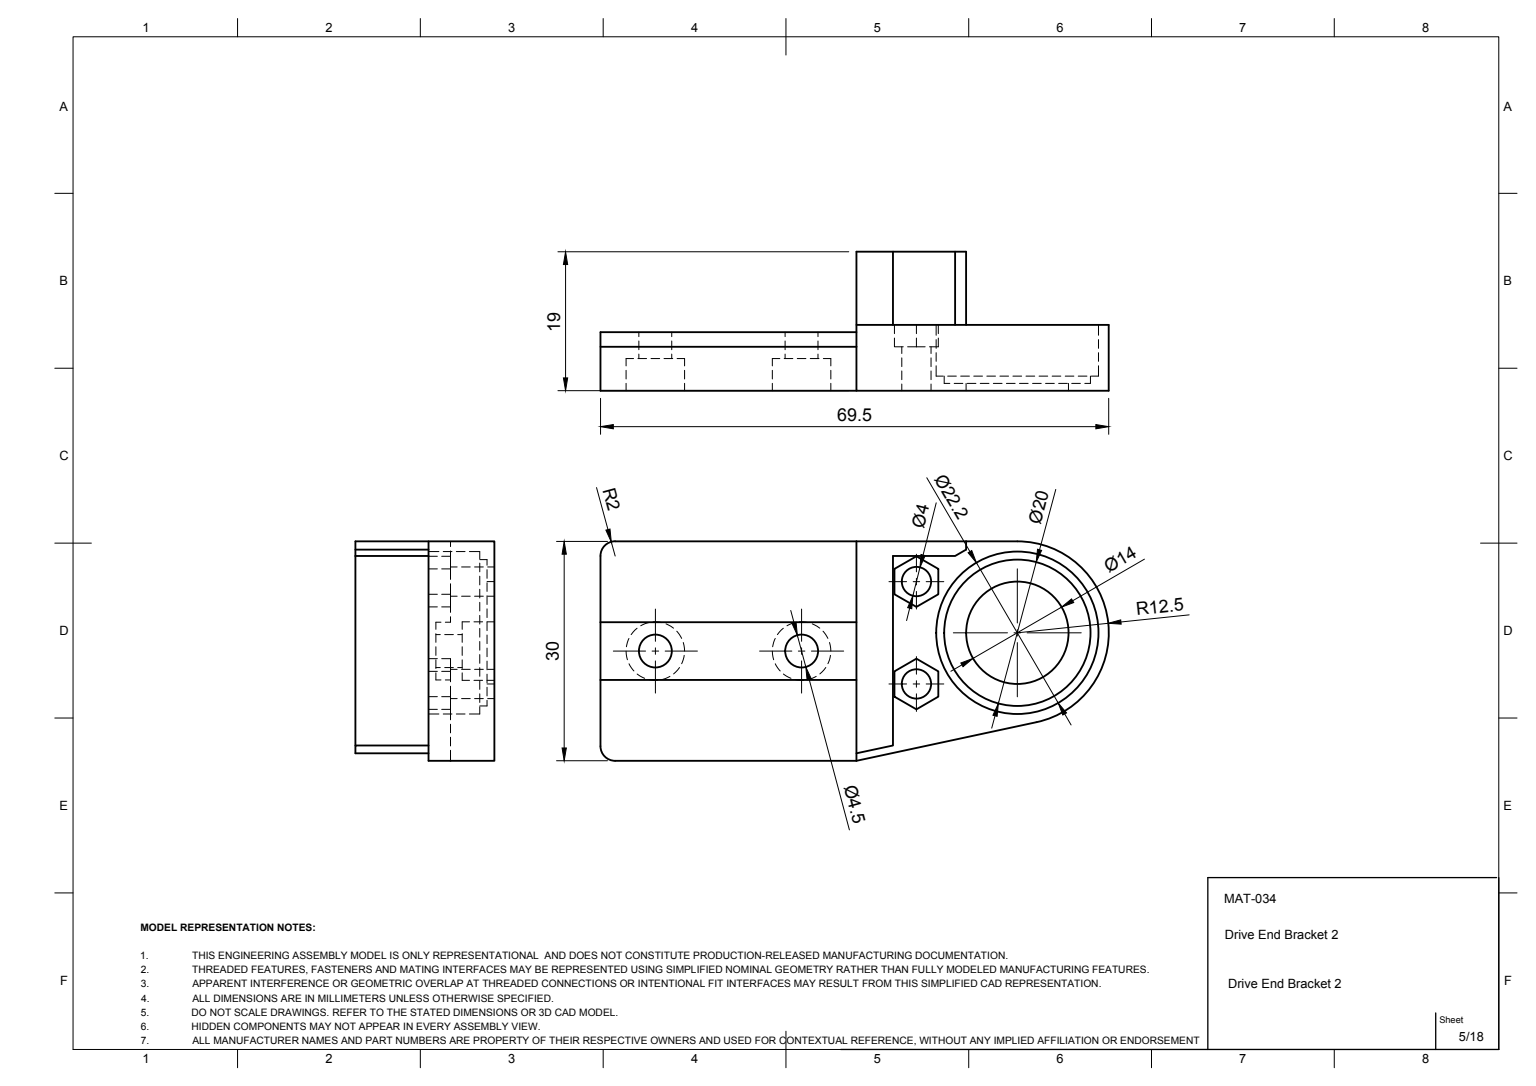
ISO-10303-21;
HEADER;
/* Generated by software containing ST-Developer
 * from STEP Tools, Inc. (www.steptools.com) 
 */

FILE_DESCRIPTION(
/* description */ ('STEP AP214'),
/* implementation_level */ '2;1');

FILE_NAME(
/* name */ 'Drive End Bracket 2.step',
/* time_stamp */ '2026-11-14T09:24:36-08:00',
/* author */ (''),
/* organization */ (''),
/* preprocessor_version */ 'ST-DEVELOPER v20.2',
/* originating_system */ 'Autodesk Translation Framework v15.17.0.0',
/* authorisation */ '');

FILE_SCHEMA (('AUTOMOTIVE_DESIGN { 1 0 10303 214 3 1 1 }'));
ENDSEC;

DATA;
#10=MECHANICAL_DESIGN_GEOMETRIC_PRESENTATION_REPRESENTATION('',(#204),#18867);
#172=SHAPE_REPRESENTATION_RELATIONSHIP('SRR','None',#18936,#188);
#188=ADVANCED_BREP_SHAPE_REPRESENTATION('',(#228),#18852);
#204=STYLED_ITEM('',(#19024),#228);
#228=MANIFOLD_SOLID_BREP('Body1',#10959);
#267=FACE_BOUND('',#1398,.T.);
#268=FACE_BOUND('',#1399,.T.);
#269=FACE_BOUND('',#1400,.T.);
#270=FACE_BOUND('',#1407,.T.);
#271=FACE_BOUND('',#1408,.T.);
#272=FACE_BOUND('',#1409,.T.);
#273=FACE_BOUND('',#1410,.T.);
#274=FACE_BOUND('',#1411,.T.);
#275=FACE_BOUND('',#1413,.T.);
#276=FACE_BOUND('',#1415,.T.);
#277=FACE_BOUND('',#1422,.T.);
#278=FACE_BOUND('',#1424,.T.);
#279=FACE_BOUND('',#1432,.T.);
#280=FACE_BOUND('',#1440,.T.);
#281=FACE_BOUND('',#1445,.T.);
#282=FACE_BOUND('',#1446,.T.);
#417=PLANE('',#11261);
#418=PLANE('',#11262);
#419=PLANE('',#11264);
#420=PLANE('',#11266);
#421=PLANE('',#11268);
#422=PLANE('',#11271);
#423=PLANE('',#11272);
#424=PLANE('',#11273);
#425=PLANE('',#11274);
#426=PLANE('',#11277);
#427=PLANE('',#11278);
#428=PLANE('',#11279);
#429=PLANE('',#11280);
#430=PLANE('',#11281);
#431=PLANE('',#11284);
#432=PLANE('',#11285);
#433=PLANE('',#11286);
#434=PLANE('',#11287);
#435=PLANE('',#11288);
#436=PLANE('',#11289);
#437=PLANE('',#11290);
#438=PLANE('',#11291);
#439=PLANE('',#11292);
#440=PLANE('',#11293);
#441=PLANE('',#11294);
#442=PLANE('',#11295);
#443=PLANE('',#11296);
#444=PLANE('',#11297);
#445=PLANE('',#11298);
#446=PLANE('',#11299);
#447=PLANE('',#11300);
#448=PLANE('',#11301);
#449=PLANE('',#11302);
#450=PLANE('',#11303);
#451=PLANE('',#11304);
#452=PLANE('',#11305);
#773=FACE_OUTER_BOUND('',#1385,.T.);
#774=FACE_OUTER_BOUND('',#1386,.T.);
#775=FACE_OUTER_BOUND('',#1387,.T.);
#776=FACE_OUTER_BOUND('',#1388,.T.);
#777=FACE_OUTER_BOUND('',#1389,.T.);
#778=FACE_OUTER_BOUND('',#1390,.T.);
#779=FACE_OUTER_BOUND('',#1391,.T.);
#780=FACE_OUTER_BOUND('',#1392,.T.);
#781=FACE_OUTER_BOUND('',#1393,.T.);
#782=FACE_OUTER_BOUND('',#1394,.T.);
#783=FACE_OUTER_BOUND('',#1395,.T.);
#784=FACE_OUTER_BOUND('',#1396,.T.);
#785=FACE_OUTER_BOUND('',#1397,.T.);
#786=FACE_OUTER_BOUND('',#1401,.T.);
#787=FACE_OUTER_BOUND('',#1402,.T.);
#788=FACE_OUTER_BOUND('',#1403,.T.);
#789=FACE_OUTER_BOUND('',#1404,.T.);
#790=FACE_OUTER_BOUND('',#1405,.T.);
#791=FACE_OUTER_BOUND('',#1406,.T.);
#792=FACE_OUTER_BOUND('',#1412,.T.);
#793=FACE_OUTER_BOUND('',#1414,.T.);
#794=FACE_OUTER_BOUND('',#1416,.T.);
#795=FACE_OUTER_BOUND('',#1417,.T.);
#796=FACE_OUTER_BOUND('',#1418,.T.);
#797=FACE_OUTER_BOUND('',#1419,.T.);
#798=FACE_OUTER_BOUND('',#1420,.T.);
#799=FACE_OUTER_BOUND('',#1421,.T.);
#800=FACE_OUTER_BOUND('',#1423,.T.);
#801=FACE_OUTER_BOUND('',#1425,.T.);
#802=FACE_OUTER_BOUND('',#1426,.T.);
#803=FACE_OUTER_BOUND('',#1427,.T.);
#804=FACE_OUTER_BOUND('',#1428,.T.);
#805=FACE_OUTER_BOUND('',#1429,.T.);
#806=FACE_OUTER_BOUND('',#1430,.T.);
#807=FACE_OUTER_BOUND('',#1431,.T.);
#808=FACE_OUTER_BOUND('',#1433,.T.);
#809=FACE_OUTER_BOUND('',#1434,.T.);
#810=FACE_OUTER_BOUND('',#1435,.T.);
#811=FACE_OUTER_BOUND('',#1436,.T.);
#812=FACE_OUTER_BOUND('',#1437,.T.);
#813=FACE_OUTER_BOUND('',#1438,.T.);
#814=FACE_OUTER_BOUND('',#1439,.T.);
#815=FACE_OUTER_BOUND('',#1441,.T.);
#816=FACE_OUTER_BOUND('',#1442,.T.);
#817=FACE_OUTER_BOUND('',#1443,.T.);
#818=FACE_OUTER_BOUND('',#1444,.T.);
#819=FACE_OUTER_BOUND('',#1447,.T.);
#820=FACE_OUTER_BOUND('',#1448,.T.);
#1385=EDGE_LOOP('',(#7346,#7347,#7348,#7349));
#1386=EDGE_LOOP('',(#7350,#7351,#7352,#7353));
#1387=EDGE_LOOP('',(#7354,#7355,#7356,#7357));
#1388=EDGE_LOOP('',(#7358,#7359,#7360,#7361));
#1389=EDGE_LOOP('',(#7362,#7363,#7364,#7365));
#1390=EDGE_LOOP('',(#7366,#7367,#7368,#7369));
#1391=EDGE_LOOP('',(#7370,#7371,#7372,#7373));
#1392=EDGE_LOOP('',(#7374,#7375,#7376,#7377));
#1393=EDGE_LOOP('',(#7378,#7379,#7380,#7381));
#1394=EDGE_LOOP('',(#7382,#7383,#7384,#7385,#7386,#7387,#7388,#7389,#7390,
#7391));
#1395=EDGE_LOOP('',(#7392,#7393,#7394,#7395,#7396));
#1396=EDGE_LOOP('',(#7397,#7398,#7399,#7400,#7401));
#1397=EDGE_LOOP('',(#7402,#7403,#7404,#7405,#7406,#7407,#7408,#7409,#7410));
#1398=EDGE_LOOP('',(#7411,#7412,#7413,#7414,#7415,#7416));
#1399=EDGE_LOOP('',(#7417,#7418,#7419,#7420,#7421,#7422));
#1400=EDGE_LOOP('',(#7423));
#1401=EDGE_LOOP('',(#7424,#7425,#7426,#7427,#7428));
#1402=EDGE_LOOP('',(#7429,#7430,#7431,#7432));
#1403=EDGE_LOOP('',(#7433,#7434,#7435,#7436,#7437,#7438,#7439,#7440));
#1404=EDGE_LOOP('',(#7441,#7442,#7443,#7444,#7445,#7446,#7447,#7448));
#1405=EDGE_LOOP('',(#7449,#7450,#7451,#7452));
#1406=EDGE_LOOP('',(#7453,#7454,#7455,#7456,#7457,#7458,#7459));
#1407=EDGE_LOOP('',(#7460));
#1408=EDGE_LOOP('',(#7461));
#1409=EDGE_LOOP('',(#7462));
#1410=EDGE_LOOP('',(#7463));
#1411=EDGE_LOOP('',(#7464));
#1412=EDGE_LOOP('',(#7465));
#1413=EDGE_LOOP('',(#7466));
#1414=EDGE_LOOP('',(#7467));
#1415=EDGE_LOOP('',(#7468));
#1416=EDGE_LOOP('',(#7469,#7470,#7471,#7472));
#1417=EDGE_LOOP('',(#7473,#7474,#7475,#7476));
#1418=EDGE_LOOP('',(#7477,#7478,#7479,#7480,#7481,#7482,#7483));
#1419=EDGE_LOOP('',(#7484,#7485,#7486,#7487));
#1420=EDGE_LOOP('',(#7488,#7489,#7490,#7491));
#1421=EDGE_LOOP('',(#7492));
#1422=EDGE_LOOP('',(#7493));
#1423=EDGE_LOOP('',(#7494));
#1424=EDGE_LOOP('',(#7495));
#1425=EDGE_LOOP('',(#7496,#7497,#7498,#7499));
#1426=EDGE_LOOP('',(#7500,#7501,#7502,#7503));
#1427=EDGE_LOOP('',(#7504,#7505,#7506,#7507));
#1428=EDGE_LOOP('',(#7508,#7509,#7510,#7511));
#1429=EDGE_LOOP('',(#7512,#7513,#7514,#7515));
#1430=EDGE_LOOP('',(#7516,#7517,#7518,#7519));
#1431=EDGE_LOOP('',(#7520,#7521,#7522,#7523,#7524,#7525));
#1432=EDGE_LOOP('',(#7526));
#1433=EDGE_LOOP('',(#7527,#7528,#7529,#7530));
#1434=EDGE_LOOP('',(#7531,#7532,#7533,#7534));
#1435=EDGE_LOOP('',(#7535,#7536,#7537,#7538));
#1436=EDGE_LOOP('',(#7539,#7540,#7541,#7542));
#1437=EDGE_LOOP('',(#7543,#7544,#7545,#7546));
#1438=EDGE_LOOP('',(#7547,#7548,#7549,#7550));
#1439=EDGE_LOOP('',(#7551,#7552,#7553,#7554,#7555,#7556));
#1440=EDGE_LOOP('',(#7557));
#1441=EDGE_LOOP('',(#7558,#7559,#7560,#7561));
#1442=EDGE_LOOP('',(#7562,#7563,#7564,#7565));
#1443=EDGE_LOOP('',(#7566,#7567,#7568,#7569));
#1444=EDGE_LOOP('',(#7570,#7571,#7572,#7573));
#1445=EDGE_LOOP('',(#7574));
#1446=EDGE_LOOP('',(#7575));
#1447=EDGE_LOOP('',(#7576,#7577,#7578,#7579));
#1448=EDGE_LOOP('',(#7580,#7581,#7582,#7583));
#2142=LINE('',#15858,#3156);
#2143=LINE('',#15864,#3157);
#2144=LINE('',#15870,#3158);
#2145=LINE('',#15876,#3159);
#2146=LINE('',#15882,#3160);
#2147=LINE('',#15888,#3161);
#2148=LINE('',#15894,#3162);
#2149=LINE('',#15900,#3163);
#2150=LINE('',#15906,#3164);
#2151=LINE('',#15911,#3165);
#2152=LINE('',#15913,#3166);
#2153=LINE('',#15915,#3167);
#2154=LINE('',#15917,#3168);
#2155=LINE('',#15919,#3169);
#2156=LINE('',#15921,#3170);
#2157=LINE('',#15923,#3171);
#2158=LINE('',#15925,#3172);
#2159=LINE('',#15927,#3173);
#2160=LINE('',#15928,#3174);
#2161=LINE('',#15931,#3175);
#2162=LINE('',#15933,#3176);
#2163=LINE('',#15936,#3177);
#2164=LINE('',#15939,#3178);
#2165=LINE('',#15941,#3179);
#2166=LINE('',#15944,#3180);
#2167=LINE('',#15948,#3181);
#2168=LINE('',#15950,#3182);
#2169=LINE('',#15951,#3183);
#2170=LINE('',#15953,#3184);
#2171=LINE('',#15957,#3185);
#2172=LINE('',#15959,#3186);
#2173=LINE('',#15960,#3187);
#2174=LINE('',#15963,#3188);
#2175=LINE('',#15965,#3189);
#2176=LINE('',#15967,#3190);
#2177=LINE('',#15969,#3191);
#2178=LINE('',#15971,#3192);
#2179=LINE('',#15972,#3193);
#2180=LINE('',#15975,#3194);
#2181=LINE('',#15977,#3195);
#2182=LINE('',#15979,#3196);
#2183=LINE('',#15981,#3197);
#2184=LINE('',#15983,#3198);
#2185=LINE('',#15984,#3199);
#2186=LINE('',#15987,#3200);
#2187=LINE('',#15989,#3201);
#2188=LINE('',#15990,#3202);
#2189=LINE('',#15994,#3203);
#2190=LINE('',#15997,#3204);
#2191=LINE('',#15998,#3205);
#2192=LINE('',#16000,#3206);
#2193=LINE('',#16001,#3207);
#2194=LINE('',#16004,#3208);
#2195=LINE('',#16006,#3209);
#2196=LINE('',#16007,#3210);
#2197=LINE('',#16009,#3211);
#2198=LINE('',#16011,#3212);
#2199=LINE('',#16012,#3213);
#2200=LINE('',#16015,#3214);
#2201=LINE('',#16016,#3215);
#2202=LINE('',#16024,#3216);
#2203=LINE('',#16025,#3217);
#2204=LINE('',#16028,#3218);
#2205=LINE('',#16029,#3219);
#2206=LINE('',#16032,#3220);
#2207=LINE('',#16034,#3221);
#2208=LINE('',#16035,#3222);
#2209=LINE('',#16042,#3223);
#2210=LINE('',#16044,#3224);
#2211=LINE('',#16045,#3225);
#2212=LINE('',#16048,#3226);
#2213=LINE('',#16049,#3227);
#2214=LINE('',#16052,#3228);
#2215=LINE('',#16053,#3229);
#2216=LINE('',#16056,#3230);
#2217=LINE('',#16057,#3231);
#2218=LINE('',#16060,#3232);
#2219=LINE('',#16061,#3233);
#2220=LINE('',#16063,#3234);
#2221=LINE('',#16067,#3235);
#2222=LINE('',#16069,#3236);
#2223=LINE('',#16070,#3237);
#2224=LINE('',#16073,#3238);
#2225=LINE('',#16074,#3239);
#2226=LINE('',#16077,#3240);
#2227=LINE('',#16078,#3241);
#2228=LINE('',#16081,#3242);
#2229=LINE('',#16082,#3243);
#2230=LINE('',#16085,#3244);
#2231=LINE('',#16086,#3245);
#2232=LINE('',#16088,#3246);
#2233=LINE('',#16091,#3247);
#2234=LINE('',#16093,#3248);
#2235=LINE('',#16096,#3249);
#2236=LINE('',#16097,#3250);
#3156=VECTOR('',#12552,2.);
#3157=VECTOR('',#12559,2.);
#3158=VECTOR('',#12566,4.);
#3159=VECTOR('',#12573,2.25);
#3160=VECTOR('',#12580,4.);
#3161=VECTOR('',#12587,2.25);
#3162=VECTOR('',#12594,7.00000000000001);
#3163=VECTOR('',#12601,10.);
#3164=VECTOR('',#12608,11.1);
#3165=VECTOR('',#12613,1000.);
#3166=VECTOR('',#12614,1000.);
#3167=VECTOR('',#12615,1000.);
#3168=VECTOR('',#12616,1000.);
#3169=VECTOR('',#12617,1000.);
#3170=VECTOR('',#12618,1000.);
#3171=VECTOR('',#12619,1000.);
#3172=VECTOR('',#12620,1000.);
#3173=VECTOR('',#12621,1000.);
#3174=VECTOR('',#12622,1000.);
#3175=VECTOR('',#12625,1000.);
#3176=VECTOR('',#12626,1000.);
#3177=VECTOR('',#12629,1000.);
#3178=VECTOR('',#12632,1000.);
#3179=VECTOR('',#12633,1000.);
#3180=VECTOR('',#12636,1000.);
#3181=VECTOR('',#12639,1000.);
#3182=VECTOR('',#12640,1000.);
#3183=VECTOR('',#12641,1000.);
#3184=VECTOR('',#12642,1000.);
#3185=VECTOR('',#12645,1000.);
#3186=VECTOR('',#12646,1000.);
#3187=VECTOR('',#12647,1000.);
#3188=VECTOR('',#12648,1000.);
#3189=VECTOR('',#12649,1000.);
#3190=VECTOR('',#12650,1000.);
#3191=VECTOR('',#12651,1000.);
#3192=VECTOR('',#12652,1000.);
#3193=VECTOR('',#12653,1000.);
#3194=VECTOR('',#12654,1000.);
#3195=VECTOR('',#12655,1000.);
#3196=VECTOR('',#12656,1000.);
#3197=VECTOR('',#12657,1000.);
#3198=VECTOR('',#12658,1000.);
#3199=VECTOR('',#12659,1000.);
#3200=VECTOR('',#12662,1000.);
#3201=VECTOR('',#12663,1000.);
#3202=VECTOR('',#12664,1000.);
#3203=VECTOR('',#12669,1000.);
#3204=VECTOR('',#12672,1000.);
#3205=VECTOR('',#12673,1000.);
#3206=VECTOR('',#12674,1000.);
#3207=VECTOR('',#12675,1000.);
#3208=VECTOR('',#12678,1000.);
#3209=VECTOR('',#12679,1000.);
#3210=VECTOR('',#12680,1000.);
#3211=VECTOR('',#12681,1000.);
#3212=VECTOR('',#12682,1000.);
#3213=VECTOR('',#12683,1000.);
#3214=VECTOR('',#12686,1000.);
#3215=VECTOR('',#12687,1000.);
#3216=VECTOR('',#12700,1000.);
#3217=VECTOR('',#12701,1000.);
#3218=VECTOR('',#12704,1000.);
#3219=VECTOR('',#12705,1000.);
#3220=VECTOR('',#12708,1000.);
#3221=VECTOR('',#12709,1000.);
#3222=VECTOR('',#12710,1000.);
#3223=VECTOR('',#12721,1000.);
#3224=VECTOR('',#12722,1000.);
#3225=VECTOR('',#12723,1000.);
#3226=VECTOR('',#12726,1000.);
#3227=VECTOR('',#12727,1000.);
#3228=VECTOR('',#12730,1000.);
#3229=VECTOR('',#12731,1000.);
#3230=VECTOR('',#12734,1000.);
#3231=VECTOR('',#12735,1000.);
#3232=VECTOR('',#12738,1000.);
#3233=VECTOR('',#12739,1000.);
#3234=VECTOR('',#12742,1000.);
#3235=VECTOR('',#12747,1000.);
#3236=VECTOR('',#12748,1000.);
#3237=VECTOR('',#12749,1000.);
#3238=VECTOR('',#12752,1000.);
#3239=VECTOR('',#12753,1000.);
#3240=VECTOR('',#12756,1000.);
#3241=VECTOR('',#12757,1000.);
#3242=VECTOR('',#12760,1000.);
#3243=VECTOR('',#12761,1000.);
#3244=VECTOR('',#12764,1000.);
#3245=VECTOR('',#12765,1000.);
#3246=VECTOR('',#12768,1000.);
#3247=VECTOR('',#12773,1000.);
#3248=VECTOR('',#12776,1000.);
#3249=VECTOR('',#12781,1000.);
#3250=VECTOR('',#12782,1000.);
#4099=CIRCLE('',#11235,2.);
#4100=CIRCLE('',#11236,2.);
#4101=CIRCLE('',#11238,2.);
#4102=CIRCLE('',#11239,2.);
#4103=CIRCLE('',#11241,4.);
#4104=CIRCLE('',#11242,4.);
#4105=CIRCLE('',#11244,2.25000000000001);
#4106=CIRCLE('',#11245,2.25);
#4107=CIRCLE('',#11247,4.);
#4108=CIRCLE('',#11248,4.);
#4109=CIRCLE('',#11250,2.25000000000001);
#4110=CIRCLE('',#11251,2.25);
#4111=CIRCLE('',#11253,7.00000000000001);
#4112=CIRCLE('',#11254,7.00000000000001);
#4113=CIRCLE('',#11256,10.);
#4114=CIRCLE('',#11257,10.);
#4115=CIRCLE('',#11259,11.1);
#4116=CIRCLE('',#11260,11.1);
#4117=CIRCLE('',#11263,2.);
#4118=CIRCLE('',#11265,2.);
#4119=CIRCLE('',#11267,12.5);
#4120=CIRCLE('',#11270,12.5);
#4121=CIRCLE('',#11275,2.);
#4122=CIRCLE('',#11276,2.);
#4653=VERTEX_POINT('',#15855);
#4654=VERTEX_POINT('',#15857);
#4655=VERTEX_POINT('',#15861);
#4656=VERTEX_POINT('',#15863);
#4657=VERTEX_POINT('',#15867);
#4658=VERTEX_POINT('',#15869);
#4659=VERTEX_POINT('',#15873);
#4660=VERTEX_POINT('',#15875);
#4661=VERTEX_POINT('',#15879);
#4662=VERTEX_POINT('',#15881);
#4663=VERTEX_POINT('',#15885);
#4664=VERTEX_POINT('',#15887);
#4665=VERTEX_POINT('',#15891);
#4666=VERTEX_POINT('',#15893);
#4667=VERTEX_POINT('',#15897);
#4668=VERTEX_POINT('',#15899);
#4669=VERTEX_POINT('',#15903);
#4670=VERTEX_POINT('',#15905);
#4671=VERTEX_POINT('',#15909);
#4672=VERTEX_POINT('',#15910);
#4673=VERTEX_POINT('',#15912);
#4674=VERTEX_POINT('',#15914);
#4675=VERTEX_POINT('',#15916);
#4676=VERTEX_POINT('',#15918);
#4677=VERTEX_POINT('',#15920);
#4678=VERTEX_POINT('',#15922);
#4679=VERTEX_POINT('',#15924);
#4680=VERTEX_POINT('',#15926);
#4681=VERTEX_POINT('',#15930);
#4682=VERTEX_POINT('',#15932);
#4683=VERTEX_POINT('',#15934);
#4684=VERTEX_POINT('',#15938);
#4685=VERTEX_POINT('',#15940);
#4686=VERTEX_POINT('',#15942);
#4687=VERTEX_POINT('',#15946);
#4688=VERTEX_POINT('',#15947);
#4689=VERTEX_POINT('',#15949);
#4690=VERTEX_POINT('',#15952);
#4691=VERTEX_POINT('',#15954);
#4692=VERTEX_POINT('',#15956);
#4693=VERTEX_POINT('',#15958);
#4694=VERTEX_POINT('',#15961);
#4695=VERTEX_POINT('',#15962);
#4696=VERTEX_POINT('',#15964);
#4697=VERTEX_POINT('',#15966);
#4698=VERTEX_POINT('',#15968);
#4699=VERTEX_POINT('',#15970);
#4700=VERTEX_POINT('',#15973);
#4701=VERTEX_POINT('',#15974);
#4702=VERTEX_POINT('',#15976);
#4703=VERTEX_POINT('',#15978);
#4704=VERTEX_POINT('',#15980);
#4705=VERTEX_POINT('',#15982);
#4706=VERTEX_POINT('',#15986);
#4707=VERTEX_POINT('',#15988);
#4708=VERTEX_POINT('',#15992);
#4709=VERTEX_POINT('',#15996);
#4710=VERTEX_POINT('',#15999);
#4711=VERTEX_POINT('',#16003);
#4712=VERTEX_POINT('',#16005);
#4713=VERTEX_POINT('',#16008);
#4714=VERTEX_POINT('',#16010);
#4715=VERTEX_POINT('',#16014);
#4716=VERTEX_POINT('',#16023);
#4717=VERTEX_POINT('',#16027);
#4718=VERTEX_POINT('',#16031);
#4719=VERTEX_POINT('',#16033);
#4720=VERTEX_POINT('',#16041);
#4721=VERTEX_POINT('',#16043);
#4722=VERTEX_POINT('',#16047);
#4723=VERTEX_POINT('',#16051);
#4724=VERTEX_POINT('',#16055);
#4725=VERTEX_POINT('',#16059);
#4726=VERTEX_POINT('',#16066);
#4727=VERTEX_POINT('',#16068);
#4728=VERTEX_POINT('',#16072);
#4729=VERTEX_POINT('',#16076);
#4730=VERTEX_POINT('',#16080);
#4731=VERTEX_POINT('',#16084);
#5706=EDGE_CURVE('',#4653,#4653,#4099,.T.);
#5707=EDGE_CURVE('',#4653,#4654,#2142,.T.);
#5708=EDGE_CURVE('',#4654,#4654,#4100,.T.);
#5709=EDGE_CURVE('',#4655,#4655,#4101,.T.);
#5710=EDGE_CURVE('',#4655,#4656,#2143,.T.);
#5711=EDGE_CURVE('',#4656,#4656,#4102,.T.);
#5712=EDGE_CURVE('',#4657,#4657,#4103,.T.);
#5713=EDGE_CURVE('',#4657,#4658,#2144,.T.);
#5714=EDGE_CURVE('',#4658,#4658,#4104,.T.);
#5715=EDGE_CURVE('',#4659,#4659,#4105,.T.);
#5716=EDGE_CURVE('',#4659,#4660,#2145,.T.);
#5717=EDGE_CURVE('',#4660,#4660,#4106,.T.);
#5718=EDGE_CURVE('',#4661,#4661,#4107,.T.);
#5719=EDGE_CURVE('',#4661,#4662,#2146,.T.);
#5720=EDGE_CURVE('',#4662,#4662,#4108,.T.);
#5721=EDGE_CURVE('',#4663,#4663,#4109,.T.);
#5722=EDGE_CURVE('',#4663,#4664,#2147,.T.);
#5723=EDGE_CURVE('',#4664,#4664,#4110,.T.);
#5724=EDGE_CURVE('',#4665,#4665,#4111,.T.);
#5725=EDGE_CURVE('',#4665,#4666,#2148,.T.);
#5726=EDGE_CURVE('',#4666,#4666,#4112,.T.);
#5727=EDGE_CURVE('',#4667,#4667,#4113,.T.);
#5728=EDGE_CURVE('',#4667,#4668,#2149,.T.);
#5729=EDGE_CURVE('',#4668,#4668,#4114,.T.);
#5730=EDGE_CURVE('',#4669,#4669,#4115,.T.);
#5731=EDGE_CURVE('',#4669,#4670,#2150,.T.);
#5732=EDGE_CURVE('',#4670,#4670,#4116,.T.);
#5733=EDGE_CURVE('',#4671,#4672,#2151,.T.);
#5734=EDGE_CURVE('',#4673,#4672,#2152,.T.);
#5735=EDGE_CURVE('',#4674,#4673,#2153,.T.);
#5736=EDGE_CURVE('',#4674,#4675,#2154,.T.);
#5737=EDGE_CURVE('',#4676,#4675,#2155,.T.);
#5738=EDGE_CURVE('',#4676,#4677,#2156,.T.);
#5739=EDGE_CURVE('',#4678,#4677,#2157,.T.);
#5740=EDGE_CURVE('',#4679,#4678,#2158,.T.);
#5741=EDGE_CURVE('',#4680,#4679,#2159,.T.);
#5742=EDGE_CURVE('',#4680,#4671,#2160,.T.);
#5743=EDGE_CURVE('',#4672,#4681,#2161,.T.);
#5744=EDGE_CURVE('',#4682,#4681,#2162,.T.);
#5745=EDGE_CURVE('',#4683,#4682,#4117,.T.);
#5746=EDGE_CURVE('',#4673,#4683,#2163,.T.);
#5747=EDGE_CURVE('',#4684,#4679,#2164,.T.);
#5748=EDGE_CURVE('',#4678,#4685,#2165,.T.);
#5749=EDGE_CURVE('',#4686,#4685,#4118,.T.);
#5750=EDGE_CURVE('',#4684,#4686,#2166,.T.);
#5751=EDGE_CURVE('',#4687,#4688,#2167,.T.);
#5752=EDGE_CURVE('',#4687,#4689,#2168,.T.);
#5753=EDGE_CURVE('',#4689,#4675,#2169,.T.);
#5754=EDGE_CURVE('',#4690,#4674,#2170,.T.);
#5755=EDGE_CURVE('',#4690,#4691,#4119,.T.);
#5756=EDGE_CURVE('',#4692,#4691,#2171,.T.);
#5757=EDGE_CURVE('',#4693,#4692,#2172,.T.);
#5758=EDGE_CURVE('',#4688,#4693,#2173,.T.);
#5759=EDGE_CURVE('',#4694,#4695,#2174,.T.);
#5760=EDGE_CURVE('',#4695,#4696,#2175,.T.);
#5761=EDGE_CURVE('',#4696,#4697,#2176,.T.);
#5762=EDGE_CURVE('',#4697,#4698,#2177,.T.);
#5763=EDGE_CURVE('',#4698,#4699,#2178,.T.);
#5764=EDGE_CURVE('',#4699,#4694,#2179,.T.);
#5765=EDGE_CURVE('',#4700,#4701,#2180,.T.);
#5766=EDGE_CURVE('',#4701,#4702,#2181,.T.);
#5767=EDGE_CURVE('',#4702,#4703,#2182,.T.);
#5768=EDGE_CURVE('',#4703,#4704,#2183,.T.);
#5769=EDGE_CURVE('',#4704,#4705,#2184,.T.);
#5770=EDGE_CURVE('',#4705,#4700,#2185,.T.);
#5771=EDGE_CURVE('',#4706,#4673,#2186,.T.);
#5772=EDGE_CURVE('',#4707,#4706,#2187,.T.);
#5773=EDGE_CURVE('',#4707,#4690,#2188,.T.);
#5774=EDGE_CURVE('',#4707,#4708,#4120,.T.);
#5775=EDGE_CURVE('',#4708,#4691,#2189,.T.);
#5776=EDGE_CURVE('',#4709,#4677,#2190,.T.);
#5777=EDGE_CURVE('',#4692,#4709,#2191,.T.);
#5778=EDGE_CURVE('',#4710,#4708,#2192,.T.);
#5779=EDGE_CURVE('',#4685,#4710,#2193,.T.);
#5780=EDGE_CURVE('',#4711,#4686,#2194,.T.);
#5781=EDGE_CURVE('',#4711,#4712,#2195,.T.);
#5782=EDGE_CURVE('',#4682,#4712,#2196,.T.);
#5783=EDGE_CURVE('',#4713,#4681,#2197,.T.);
#5784=EDGE_CURVE('',#4713,#4714,#2198,.T.);
#5785=EDGE_CURVE('',#4714,#4684,#2199,.T.);
#5786=EDGE_CURVE('',#4715,#4683,#2200,.T.);
#5787=EDGE_CURVE('',#4715,#4706,#2201,.T.);
#5788=EDGE_CURVE('',#4710,#4711,#4121,.T.);
#5789=EDGE_CURVE('',#4712,#4715,#4122,.T.);
#5790=EDGE_CURVE('',#4716,#4689,#2202,.T.);
#5791=EDGE_CURVE('',#4716,#4676,#2203,.T.);
#5792=EDGE_CURVE('',#4717,#4716,#2204,.T.);
#5793=EDGE_CURVE('',#4717,#4687,#2205,.T.);
#5794=EDGE_CURVE('',#4718,#4709,#2206,.T.);
#5795=EDGE_CURVE('',#4719,#4717,#2207,.T.);
#5796=EDGE_CURVE('',#4718,#4719,#2208,.T.);
#5797=EDGE_CURVE('',#4720,#4705,#2209,.T.);
#5798=EDGE_CURVE('',#4720,#4721,#2210,.T.);
#5799=EDGE_CURVE('',#4721,#4700,#2211,.T.);
#5800=EDGE_CURVE('',#4722,#4704,#2212,.T.);
#5801=EDGE_CURVE('',#4722,#4720,#2213,.T.);
#5802=EDGE_CURVE('',#4723,#4703,#2214,.T.);
#5803=EDGE_CURVE('',#4723,#4722,#2215,.T.);
#5804=EDGE_CURVE('',#4724,#4702,#2216,.T.);
#5805=EDGE_CURVE('',#4724,#4723,#2217,.T.);
#5806=EDGE_CURVE('',#4725,#4701,#2218,.T.);
#5807=EDGE_CURVE('',#4725,#4724,#2219,.T.);
#5808=EDGE_CURVE('',#4721,#4725,#2220,.T.);
#5809=EDGE_CURVE('',#4726,#4699,#2221,.T.);
#5810=EDGE_CURVE('',#4726,#4727,#2222,.T.);
#5811=EDGE_CURVE('',#4727,#4694,#2223,.T.);
#5812=EDGE_CURVE('',#4728,#4698,#2224,.T.);
#5813=EDGE_CURVE('',#4728,#4726,#2225,.T.);
#5814=EDGE_CURVE('',#4729,#4697,#2226,.T.);
#5815=EDGE_CURVE('',#4729,#4728,#2227,.T.);
#5816=EDGE_CURVE('',#4730,#4696,#2228,.T.);
#5817=EDGE_CURVE('',#4730,#4729,#2229,.T.);
#5818=EDGE_CURVE('',#4731,#4695,#2230,.T.);
#5819=EDGE_CURVE('',#4731,#4730,#2231,.T.);
#5820=EDGE_CURVE('',#4727,#4731,#2232,.T.);
#5821=EDGE_CURVE('',#4719,#4688,#2233,.T.);
#5822=EDGE_CURVE('',#4693,#4718,#2234,.T.);
#5823=EDGE_CURVE('',#4714,#4680,#2235,.T.);
#5824=EDGE_CURVE('',#4671,#4713,#2236,.T.);
#7346=ORIENTED_EDGE('',*,*,#5706,.T.);
#7347=ORIENTED_EDGE('',*,*,#5707,.T.);
#7348=ORIENTED_EDGE('',*,*,#5708,.F.);
#7349=ORIENTED_EDGE('',*,*,#5707,.F.);
#7350=ORIENTED_EDGE('',*,*,#5709,.T.);
#7351=ORIENTED_EDGE('',*,*,#5710,.T.);
#7352=ORIENTED_EDGE('',*,*,#5711,.F.);
#7353=ORIENTED_EDGE('',*,*,#5710,.F.);
#7354=ORIENTED_EDGE('',*,*,#5712,.T.);
#7355=ORIENTED_EDGE('',*,*,#5713,.T.);
#7356=ORIENTED_EDGE('',*,*,#5714,.F.);
#7357=ORIENTED_EDGE('',*,*,#5713,.F.);
#7358=ORIENTED_EDGE('',*,*,#5715,.F.);
#7359=ORIENTED_EDGE('',*,*,#5716,.T.);
#7360=ORIENTED_EDGE('',*,*,#5717,.F.);
#7361=ORIENTED_EDGE('',*,*,#5716,.F.);
#7362=ORIENTED_EDGE('',*,*,#5718,.T.);
#7363=ORIENTED_EDGE('',*,*,#5719,.T.);
#7364=ORIENTED_EDGE('',*,*,#5720,.F.);
#7365=ORIENTED_EDGE('',*,*,#5719,.F.);
#7366=ORIENTED_EDGE('',*,*,#5721,.F.);
#7367=ORIENTED_EDGE('',*,*,#5722,.T.);
#7368=ORIENTED_EDGE('',*,*,#5723,.F.);
#7369=ORIENTED_EDGE('',*,*,#5722,.F.);
#7370=ORIENTED_EDGE('',*,*,#5724,.T.);
#7371=ORIENTED_EDGE('',*,*,#5725,.T.);
#7372=ORIENTED_EDGE('',*,*,#5726,.F.);
#7373=ORIENTED_EDGE('',*,*,#5725,.F.);
#7374=ORIENTED_EDGE('',*,*,#5727,.T.);
#7375=ORIENTED_EDGE('',*,*,#5728,.T.);
#7376=ORIENTED_EDGE('',*,*,#5729,.F.);
#7377=ORIENTED_EDGE('',*,*,#5728,.F.);
#7378=ORIENTED_EDGE('',*,*,#5730,.T.);
#7379=ORIENTED_EDGE('',*,*,#5731,.T.);
#7380=ORIENTED_EDGE('',*,*,#5732,.F.);
#7381=ORIENTED_EDGE('',*,*,#5731,.F.);
#7382=ORIENTED_EDGE('',*,*,#5733,.T.);
#7383=ORIENTED_EDGE('',*,*,#5734,.F.);
#7384=ORIENTED_EDGE('',*,*,#5735,.F.);
#7385=ORIENTED_EDGE('',*,*,#5736,.T.);
#7386=ORIENTED_EDGE('',*,*,#5737,.F.);
#7387=ORIENTED_EDGE('',*,*,#5738,.T.);
#7388=ORIENTED_EDGE('',*,*,#5739,.F.);
#7389=ORIENTED_EDGE('',*,*,#5740,.F.);
#7390=ORIENTED_EDGE('',*,*,#5741,.F.);
#7391=ORIENTED_EDGE('',*,*,#5742,.T.);
#7392=ORIENTED_EDGE('',*,*,#5743,.T.);
#7393=ORIENTED_EDGE('',*,*,#5744,.F.);
#7394=ORIENTED_EDGE('',*,*,#5745,.F.);
#7395=ORIENTED_EDGE('',*,*,#5746,.F.);
#7396=ORIENTED_EDGE('',*,*,#5734,.T.);
#7397=ORIENTED_EDGE('',*,*,#5747,.T.);
#7398=ORIENTED_EDGE('',*,*,#5740,.T.);
#7399=ORIENTED_EDGE('',*,*,#5748,.T.);
#7400=ORIENTED_EDGE('',*,*,#5749,.F.);
#7401=ORIENTED_EDGE('',*,*,#5750,.F.);
#7402=ORIENTED_EDGE('',*,*,#5751,.F.);
#7403=ORIENTED_EDGE('',*,*,#5752,.T.);
#7404=ORIENTED_EDGE('',*,*,#5753,.T.);
#7405=ORIENTED_EDGE('',*,*,#5736,.F.);
#7406=ORIENTED_EDGE('',*,*,#5754,.F.);
#7407=ORIENTED_EDGE('',*,*,#5755,.T.);
#7408=ORIENTED_EDGE('',*,*,#5756,.F.);
#7409=ORIENTED_EDGE('',*,*,#5757,.F.);
#7410=ORIENTED_EDGE('',*,*,#5758,.F.);
#7411=ORIENTED_EDGE('',*,*,#5759,.T.);
#7412=ORIENTED_EDGE('',*,*,#5760,.T.);
#7413=ORIENTED_EDGE('',*,*,#5761,.T.);
#7414=ORIENTED_EDGE('',*,*,#5762,.T.);
#7415=ORIENTED_EDGE('',*,*,#5763,.T.);
#7416=ORIENTED_EDGE('',*,*,#5764,.T.);
#7417=ORIENTED_EDGE('',*,*,#5765,.T.);
#7418=ORIENTED_EDGE('',*,*,#5766,.T.);
#7419=ORIENTED_EDGE('',*,*,#5767,.T.);
#7420=ORIENTED_EDGE('',*,*,#5768,.T.);
#7421=ORIENTED_EDGE('',*,*,#5769,.T.);
#7422=ORIENTED_EDGE('',*,*,#5770,.T.);
#7423=ORIENTED_EDGE('',*,*,#5732,.T.);
#7424=ORIENTED_EDGE('',*,*,#5754,.T.);
#7425=ORIENTED_EDGE('',*,*,#5735,.T.);
#7426=ORIENTED_EDGE('',*,*,#5771,.F.);
#7427=ORIENTED_EDGE('',*,*,#5772,.F.);
#7428=ORIENTED_EDGE('',*,*,#5773,.T.);
#7429=ORIENTED_EDGE('',*,*,#5755,.F.);
#7430=ORIENTED_EDGE('',*,*,#5773,.F.);
#7431=ORIENTED_EDGE('',*,*,#5774,.T.);
#7432=ORIENTED_EDGE('',*,*,#5775,.T.);
#7433=ORIENTED_EDGE('',*,*,#5748,.F.);
#7434=ORIENTED_EDGE('',*,*,#5739,.T.);
#7435=ORIENTED_EDGE('',*,*,#5776,.F.);
#7436=ORIENTED_EDGE('',*,*,#5777,.F.);
#7437=ORIENTED_EDGE('',*,*,#5756,.T.);
#7438=ORIENTED_EDGE('',*,*,#5775,.F.);
#7439=ORIENTED_EDGE('',*,*,#5778,.F.);
#7440=ORIENTED_EDGE('',*,*,#5779,.F.);
#7441=ORIENTED_EDGE('',*,*,#5780,.F.);
#7442=ORIENTED_EDGE('',*,*,#5781,.T.);
#7443=ORIENTED_EDGE('',*,*,#5782,.F.);
#7444=ORIENTED_EDGE('',*,*,#5744,.T.);
#7445=ORIENTED_EDGE('',*,*,#5783,.F.);
#7446=ORIENTED_EDGE('',*,*,#5784,.T.);
#7447=ORIENTED_EDGE('',*,*,#5785,.T.);
#7448=ORIENTED_EDGE('',*,*,#5750,.T.);
#7449=ORIENTED_EDGE('',*,*,#5786,.F.);
#7450=ORIENTED_EDGE('',*,*,#5787,.T.);
#7451=ORIENTED_EDGE('',*,*,#5771,.T.);
#7452=ORIENTED_EDGE('',*,*,#5746,.T.);
#7453=ORIENTED_EDGE('',*,*,#5781,.F.);
#7454=ORIENTED_EDGE('',*,*,#5788,.F.);
#7455=ORIENTED_EDGE('',*,*,#5778,.T.);
#7456=ORIENTED_EDGE('',*,*,#5774,.F.);
#7457=ORIENTED_EDGE('',*,*,#5772,.T.);
#7458=ORIENTED_EDGE('',*,*,#5787,.F.);
#7459=ORIENTED_EDGE('',*,*,#5789,.F.);
#7460=ORIENTED_EDGE('',*,*,#5706,.F.);
#7461=ORIENTED_EDGE('',*,*,#5709,.F.);
#7462=ORIENTED_EDGE('',*,*,#5714,.T.);
#7463=ORIENTED_EDGE('',*,*,#5720,.T.);
#7464=ORIENTED_EDGE('',*,*,#5724,.F.);
#7465=ORIENTED_EDGE('',*,*,#5730,.F.);
#7466=ORIENTED_EDGE('',*,*,#5729,.T.);
#7467=ORIENTED_EDGE('',*,*,#5727,.F.);
#7468=ORIENTED_EDGE('',*,*,#5726,.T.);
#7469=ORIENTED_EDGE('',*,*,#5753,.F.);
#7470=ORIENTED_EDGE('',*,*,#5790,.F.);
#7471=ORIENTED_EDGE('',*,*,#5791,.T.);
#7472=ORIENTED_EDGE('',*,*,#5737,.T.);
#7473=ORIENTED_EDGE('',*,*,#5792,.T.);
#7474=ORIENTED_EDGE('',*,*,#5790,.T.);
#7475=ORIENTED_EDGE('',*,*,#5752,.F.);
#7476=ORIENTED_EDGE('',*,*,#5793,.F.);
#7477=ORIENTED_EDGE('',*,*,#5794,.T.);
#7478=ORIENTED_EDGE('',*,*,#5776,.T.);
#7479=ORIENTED_EDGE('',*,*,#5738,.F.);
#7480=ORIENTED_EDGE('',*,*,#5791,.F.);
#7481=ORIENTED_EDGE('',*,*,#5792,.F.);
#7482=ORIENTED_EDGE('',*,*,#5795,.F.);
#7483=ORIENTED_EDGE('',*,*,#5796,.F.);
#7484=ORIENTED_EDGE('',*,*,#5745,.T.);
#7485=ORIENTED_EDGE('',*,*,#5782,.T.);
#7486=ORIENTED_EDGE('',*,*,#5789,.T.);
#7487=ORIENTED_EDGE('',*,*,#5786,.T.);
#7488=ORIENTED_EDGE('',*,*,#5749,.T.);
#7489=ORIENTED_EDGE('',*,*,#5779,.T.);
#7490=ORIENTED_EDGE('',*,*,#5788,.T.);
#7491=ORIENTED_EDGE('',*,*,#5780,.T.);
#7492=ORIENTED_EDGE('',*,*,#5718,.F.);
#7493=ORIENTED_EDGE('',*,*,#5723,.T.);
#7494=ORIENTED_EDGE('',*,*,#5712,.F.);
#7495=ORIENTED_EDGE('',*,*,#5717,.T.);
#7496=ORIENTED_EDGE('',*,*,#5770,.F.);
#7497=ORIENTED_EDGE('',*,*,#5797,.F.);
#7498=ORIENTED_EDGE('',*,*,#5798,.T.);
#7499=ORIENTED_EDGE('',*,*,#5799,.T.);
#7500=ORIENTED_EDGE('',*,*,#5769,.F.);
#7501=ORIENTED_EDGE('',*,*,#5800,.F.);
#7502=ORIENTED_EDGE('',*,*,#5801,.T.);
#7503=ORIENTED_EDGE('',*,*,#5797,.T.);
#7504=ORIENTED_EDGE('',*,*,#5768,.F.);
#7505=ORIENTED_EDGE('',*,*,#5802,.F.);
#7506=ORIENTED_EDGE('',*,*,#5803,.T.);
#7507=ORIENTED_EDGE('',*,*,#5800,.T.);
#7508=ORIENTED_EDGE('',*,*,#5767,.F.);
#7509=ORIENTED_EDGE('',*,*,#5804,.F.);
#7510=ORIENTED_EDGE('',*,*,#5805,.T.);
#7511=ORIENTED_EDGE('',*,*,#5802,.T.);
#7512=ORIENTED_EDGE('',*,*,#5766,.F.);
#7513=ORIENTED_EDGE('',*,*,#5806,.F.);
#7514=ORIENTED_EDGE('',*,*,#5807,.T.);
#7515=ORIENTED_EDGE('',*,*,#5804,.T.);
#7516=ORIENTED_EDGE('',*,*,#5765,.F.);
#7517=ORIENTED_EDGE('',*,*,#5799,.F.);
#7518=ORIENTED_EDGE('',*,*,#5808,.T.);
#7519=ORIENTED_EDGE('',*,*,#5806,.T.);
#7520=ORIENTED_EDGE('',*,*,#5798,.F.);
#7521=ORIENTED_EDGE('',*,*,#5801,.F.);
#7522=ORIENTED_EDGE('',*,*,#5803,.F.);
#7523=ORIENTED_EDGE('',*,*,#5805,.F.);
#7524=ORIENTED_EDGE('',*,*,#5807,.F.);
#7525=ORIENTED_EDGE('',*,*,#5808,.F.);
#7526=ORIENTED_EDGE('',*,*,#5711,.T.);
#7527=ORIENTED_EDGE('',*,*,#5764,.F.);
#7528=ORIENTED_EDGE('',*,*,#5809,.F.);
#7529=ORIENTED_EDGE('',*,*,#5810,.T.);
#7530=ORIENTED_EDGE('',*,*,#5811,.T.);
#7531=ORIENTED_EDGE('',*,*,#5763,.F.);
#7532=ORIENTED_EDGE('',*,*,#5812,.F.);
#7533=ORIENTED_EDGE('',*,*,#5813,.T.);
#7534=ORIENTED_EDGE('',*,*,#5809,.T.);
#7535=ORIENTED_EDGE('',*,*,#5762,.F.);
#7536=ORIENTED_EDGE('',*,*,#5814,.F.);
#7537=ORIENTED_EDGE('',*,*,#5815,.T.);
#7538=ORIENTED_EDGE('',*,*,#5812,.T.);
#7539=ORIENTED_EDGE('',*,*,#5761,.F.);
#7540=ORIENTED_EDGE('',*,*,#5816,.F.);
#7541=ORIENTED_EDGE('',*,*,#5817,.T.);
#7542=ORIENTED_EDGE('',*,*,#5814,.T.);
#7543=ORIENTED_EDGE('',*,*,#5760,.F.);
#7544=ORIENTED_EDGE('',*,*,#5818,.F.);
#7545=ORIENTED_EDGE('',*,*,#5819,.T.);
#7546=ORIENTED_EDGE('',*,*,#5816,.T.);
#7547=ORIENTED_EDGE('',*,*,#5759,.F.);
#7548=ORIENTED_EDGE('',*,*,#5811,.F.);
#7549=ORIENTED_EDGE('',*,*,#5820,.T.);
#7550=ORIENTED_EDGE('',*,*,#5818,.T.);
#7551=ORIENTED_EDGE('',*,*,#5810,.F.);
#7552=ORIENTED_EDGE('',*,*,#5813,.F.);
#7553=ORIENTED_EDGE('',*,*,#5815,.F.);
#7554=ORIENTED_EDGE('',*,*,#5817,.F.);
#7555=ORIENTED_EDGE('',*,*,#5819,.F.);
#7556=ORIENTED_EDGE('',*,*,#5820,.F.);
#7557=ORIENTED_EDGE('',*,*,#5708,.T.);
#7558=ORIENTED_EDGE('',*,*,#5795,.T.);
#7559=ORIENTED_EDGE('',*,*,#5793,.T.);
#7560=ORIENTED_EDGE('',*,*,#5751,.T.);
#7561=ORIENTED_EDGE('',*,*,#5821,.F.);
#7562=ORIENTED_EDGE('',*,*,#5757,.T.);
#7563=ORIENTED_EDGE('',*,*,#5777,.T.);
#7564=ORIENTED_EDGE('',*,*,#5794,.F.);
#7565=ORIENTED_EDGE('',*,*,#5822,.F.);
#7566=ORIENTED_EDGE('',*,*,#5758,.T.);
#7567=ORIENTED_EDGE('',*,*,#5822,.T.);
#7568=ORIENTED_EDGE('',*,*,#5796,.T.);
#7569=ORIENTED_EDGE('',*,*,#5821,.T.);
#7570=ORIENTED_EDGE('',*,*,#5742,.F.);
#7571=ORIENTED_EDGE('',*,*,#5823,.F.);
#7572=ORIENTED_EDGE('',*,*,#5784,.F.);
#7573=ORIENTED_EDGE('',*,*,#5824,.F.);
#7574=ORIENTED_EDGE('',*,*,#5721,.T.);
#7575=ORIENTED_EDGE('',*,*,#5715,.T.);
#7576=ORIENTED_EDGE('',*,*,#5743,.F.);
#7577=ORIENTED_EDGE('',*,*,#5733,.F.);
#7578=ORIENTED_EDGE('',*,*,#5824,.T.);
#7579=ORIENTED_EDGE('',*,*,#5783,.T.);
#7580=ORIENTED_EDGE('',*,*,#5747,.F.);
#7581=ORIENTED_EDGE('',*,*,#5785,.F.);
#7582=ORIENTED_EDGE('',*,*,#5823,.T.);
#7583=ORIENTED_EDGE('',*,*,#5741,.T.);
#10162=CYLINDRICAL_SURFACE('',#11234,2.);
#10163=CYLINDRICAL_SURFACE('',#11237,2.);
#10164=CYLINDRICAL_SURFACE('',#11240,4.);
#10165=CYLINDRICAL_SURFACE('',#11243,2.25);
#10166=CYLINDRICAL_SURFACE('',#11246,4.);
#10167=CYLINDRICAL_SURFACE('',#11249,2.25);
#10168=CYLINDRICAL_SURFACE('',#11252,7.00000000000001);
#10169=CYLINDRICAL_SURFACE('',#11255,10.);
#10170=CYLINDRICAL_SURFACE('',#11258,11.1);
#10171=CYLINDRICAL_SURFACE('',#11269,12.5);
#10172=CYLINDRICAL_SURFACE('',#11282,2.);
#10173=CYLINDRICAL_SURFACE('',#11283,2.);
#10410=ADVANCED_FACE('',(#773),#10162,.F.);
#10411=ADVANCED_FACE('',(#774),#10163,.F.);
#10412=ADVANCED_FACE('',(#775),#10164,.F.);
#10413=ADVANCED_FACE('',(#776),#10165,.F.);
#10414=ADVANCED_FACE('',(#777),#10166,.F.);
#10415=ADVANCED_FACE('',(#778),#10167,.F.);
#10416=ADVANCED_FACE('',(#779),#10168,.F.);
#10417=ADVANCED_FACE('',(#780),#10169,.F.);
#10418=ADVANCED_FACE('',(#781),#10170,.F.);
#10419=ADVANCED_FACE('',(#782),#417,.F.);
#10420=ADVANCED_FACE('',(#783),#418,.F.);
#10421=ADVANCED_FACE('',(#784),#419,.F.);
#10422=ADVANCED_FACE('',(#785,#267,#268,#269),#420,.F.);
#10423=ADVANCED_FACE('',(#786),#421,.T.);
#10424=ADVANCED_FACE('',(#787),#10171,.T.);
#10425=ADVANCED_FACE('',(#788),#422,.T.);
#10426=ADVANCED_FACE('',(#789),#423,.F.);
#10427=ADVANCED_FACE('',(#790),#424,.F.);
#10428=ADVANCED_FACE('',(#791,#270,#271,#272,#273,#274),#425,.T.);
#10429=ADVANCED_FACE('',(#792,#275),#426,.T.);
#10430=ADVANCED_FACE('',(#793,#276),#427,.T.);
#10431=ADVANCED_FACE('',(#794),#428,.F.);
#10432=ADVANCED_FACE('',(#795),#429,.F.);
#10433=ADVANCED_FACE('',(#796),#430,.T.);
#10434=ADVANCED_FACE('',(#797),#10172,.T.);
#10435=ADVANCED_FACE('',(#798),#10173,.T.);
#10436=ADVANCED_FACE('',(#799,#277),#431,.F.);
#10437=ADVANCED_FACE('',(#800,#278),#432,.F.);
#10438=ADVANCED_FACE('',(#801),#433,.F.);
#10439=ADVANCED_FACE('',(#802),#434,.F.);
#10440=ADVANCED_FACE('',(#803),#435,.F.);
#10441=ADVANCED_FACE('',(#804),#436,.F.);
#10442=ADVANCED_FACE('',(#805),#437,.F.);
#10443=ADVANCED_FACE('',(#806),#438,.F.);
#10444=ADVANCED_FACE('',(#807,#279),#439,.F.);
#10445=ADVANCED_FACE('',(#808),#440,.F.);
#10446=ADVANCED_FACE('',(#809),#441,.F.);
#10447=ADVANCED_FACE('',(#810),#442,.F.);
#10448=ADVANCED_FACE('',(#811),#443,.F.);
#10449=ADVANCED_FACE('',(#812),#444,.F.);
#10450=ADVANCED_FACE('',(#813),#445,.F.);
#10451=ADVANCED_FACE('',(#814,#280),#446,.T.);
#10452=ADVANCED_FACE('',(#815),#447,.T.);
#10453=ADVANCED_FACE('',(#816),#448,.T.);
#10454=ADVANCED_FACE('',(#817),#449,.F.);
#10455=ADVANCED_FACE('',(#818,#281,#282),#450,.T.);
#10456=ADVANCED_FACE('',(#819),#451,.F.);
#10457=ADVANCED_FACE('',(#820),#452,.F.);
#10959=CLOSED_SHELL('',(#10410,#10411,#10412,#10413,#10414,#10415,#10416,
#10417,#10418,#10419,#10420,#10421,#10422,#10423,#10424,#10425,#10426,#10427,
#10428,#10429,#10430,#10431,#10432,#10433,#10434,#10435,#10436,#10437,#10438,
#10439,#10440,#10441,#10442,#10443,#10444,#10445,#10446,#10447,#10448,#10449,
#10450,#10451,#10452,#10453,#10454,#10455,#10456,#10457));
#11233=AXIS2_PLACEMENT_3D('',#15853,#12546,#12547);
#11234=AXIS2_PLACEMENT_3D('',#15854,#12548,#12549);
#11235=AXIS2_PLACEMENT_3D('',#15856,#12550,#12551);
#11236=AXIS2_PLACEMENT_3D('',#15859,#12553,#12554);
#11237=AXIS2_PLACEMENT_3D('',#15860,#12555,#12556);
#11238=AXIS2_PLACEMENT_3D('',#15862,#12557,#12558);
#11239=AXIS2_PLACEMENT_3D('',#15865,#12560,#12561);
#11240=AXIS2_PLACEMENT_3D('',#15866,#12562,#12563);
#11241=AXIS2_PLACEMENT_3D('',#15868,#12564,#12565);
#11242=AXIS2_PLACEMENT_3D('',#15871,#12567,#12568);
#11243=AXIS2_PLACEMENT_3D('',#15872,#12569,#12570);
#11244=AXIS2_PLACEMENT_3D('',#15874,#12571,#12572);
#11245=AXIS2_PLACEMENT_3D('',#15877,#12574,#12575);
#11246=AXIS2_PLACEMENT_3D('',#15878,#12576,#12577);
#11247=AXIS2_PLACEMENT_3D('',#15880,#12578,#12579);
#11248=AXIS2_PLACEMENT_3D('',#15883,#12581,#12582);
#11249=AXIS2_PLACEMENT_3D('',#15884,#12583,#12584);
#11250=AXIS2_PLACEMENT_3D('',#15886,#12585,#12586);
#11251=AXIS2_PLACEMENT_3D('',#15889,#12588,#12589);
#11252=AXIS2_PLACEMENT_3D('',#15890,#12590,#12591);
#11253=AXIS2_PLACEMENT_3D('',#15892,#12592,#12593);
#11254=AXIS2_PLACEMENT_3D('',#15895,#12595,#12596);
#11255=AXIS2_PLACEMENT_3D('',#15896,#12597,#12598);
#11256=AXIS2_PLACEMENT_3D('',#15898,#12599,#12600);
#11257=AXIS2_PLACEMENT_3D('',#15901,#12602,#12603);
#11258=AXIS2_PLACEMENT_3D('',#15902,#12604,#12605);
#11259=AXIS2_PLACEMENT_3D('',#15904,#12606,#12607);
#11260=AXIS2_PLACEMENT_3D('',#15907,#12609,#12610);
#11261=AXIS2_PLACEMENT_3D('',#15908,#12611,#12612);
#11262=AXIS2_PLACEMENT_3D('',#15929,#12623,#12624);
#11263=AXIS2_PLACEMENT_3D('',#15935,#12627,#12628);
#11264=AXIS2_PLACEMENT_3D('',#15937,#12630,#12631);
#11265=AXIS2_PLACEMENT_3D('',#15943,#12634,#12635);
#11266=AXIS2_PLACEMENT_3D('',#15945,#12637,#12638);
#11267=AXIS2_PLACEMENT_3D('',#15955,#12643,#12644);
#11268=AXIS2_PLACEMENT_3D('',#15985,#12660,#12661);
#11269=AXIS2_PLACEMENT_3D('',#15991,#12665,#12666);
#11270=AXIS2_PLACEMENT_3D('',#15993,#12667,#12668);
#11271=AXIS2_PLACEMENT_3D('',#15995,#12670,#12671);
#11272=AXIS2_PLACEMENT_3D('',#16002,#12676,#12677);
#11273=AXIS2_PLACEMENT_3D('',#16013,#12684,#12685);
#11274=AXIS2_PLACEMENT_3D('',#16017,#12688,#12689);
#11275=AXIS2_PLACEMENT_3D('',#16018,#12690,#12691);
#11276=AXIS2_PLACEMENT_3D('',#16019,#12692,#12693);
#11277=AXIS2_PLACEMENT_3D('',#16020,#12694,#12695);
#11278=AXIS2_PLACEMENT_3D('',#16021,#12696,#12697);
#11279=AXIS2_PLACEMENT_3D('',#16022,#12698,#12699);
#11280=AXIS2_PLACEMENT_3D('',#16026,#12702,#12703);
#11281=AXIS2_PLACEMENT_3D('',#16030,#12706,#12707);
#11282=AXIS2_PLACEMENT_3D('',#16036,#12711,#12712);
#11283=AXIS2_PLACEMENT_3D('',#16037,#12713,#12714);
#11284=AXIS2_PLACEMENT_3D('',#16038,#12715,#12716);
#11285=AXIS2_PLACEMENT_3D('',#16039,#12717,#12718);
#11286=AXIS2_PLACEMENT_3D('',#16040,#12719,#12720);
#11287=AXIS2_PLACEMENT_3D('',#16046,#12724,#12725);
#11288=AXIS2_PLACEMENT_3D('',#16050,#12728,#12729);
#11289=AXIS2_PLACEMENT_3D('',#16054,#12732,#12733);
#11290=AXIS2_PLACEMENT_3D('',#16058,#12736,#12737);
#11291=AXIS2_PLACEMENT_3D('',#16062,#12740,#12741);
#11292=AXIS2_PLACEMENT_3D('',#16064,#12743,#12744);
#11293=AXIS2_PLACEMENT_3D('',#16065,#12745,#12746);
#11294=AXIS2_PLACEMENT_3D('',#16071,#12750,#12751);
#11295=AXIS2_PLACEMENT_3D('',#16075,#12754,#12755);
#11296=AXIS2_PLACEMENT_3D('',#16079,#12758,#12759);
#11297=AXIS2_PLACEMENT_3D('',#16083,#12762,#12763);
#11298=AXIS2_PLACEMENT_3D('',#16087,#12766,#12767);
#11299=AXIS2_PLACEMENT_3D('',#16089,#12769,#12770);
#11300=AXIS2_PLACEMENT_3D('',#16090,#12771,#12772);
#11301=AXIS2_PLACEMENT_3D('',#16092,#12774,#12775);
#11302=AXIS2_PLACEMENT_3D('',#16094,#12777,#12778);
#11303=AXIS2_PLACEMENT_3D('',#16095,#12779,#12780);
#11304=AXIS2_PLACEMENT_3D('',#16098,#12783,#12784);
#11305=AXIS2_PLACEMENT_3D('',#16099,#12785,#12786);
#12546=DIRECTION('axis',(0.,0.,1.));
#12547=DIRECTION('refdir',(1.,0.,0.));
#12548=DIRECTION('center_axis',(0.,0.,1.));
#12549=DIRECTION('ref_axis',(-1.,0.,0.));
#12550=DIRECTION('center_axis',(0.,0.,-1.));
#12551=DIRECTION('ref_axis',(-1.,0.,0.));
#12552=DIRECTION('',(0.,0.,1.));
#12553=DIRECTION('center_axis',(0.,0.,-1.));
#12554=DIRECTION('ref_axis',(-1.,0.,0.));
#12555=DIRECTION('center_axis',(0.,0.,1.));
#12556=DIRECTION('ref_axis',(-1.,0.,0.));
#12557=DIRECTION('center_axis',(0.,0.,-1.));
#12558=DIRECTION('ref_axis',(-1.,0.,0.));
#12559=DIRECTION('',(0.,0.,1.));
#12560=DIRECTION('center_axis',(0.,0.,-1.));
#12561=DIRECTION('ref_axis',(-1.,0.,0.));
#12562=DIRECTION('center_axis',(0.,0.,-1.));
#12563=DIRECTION('ref_axis',(1.,0.,0.));
#12564=DIRECTION('center_axis',(0.,0.,1.));
#12565=DIRECTION('ref_axis',(1.,0.,0.));
#12566=DIRECTION('',(0.,0.,-1.));
#12567=DIRECTION('center_axis',(0.,0.,1.));
#12568=DIRECTION('ref_axis',(1.,0.,0.));
#12569=DIRECTION('center_axis',(0.,0.,-1.));
#12570=DIRECTION('ref_axis',(1.,0.,0.));
#12571=DIRECTION('center_axis',(0.,1.15648231731787E-16,-1.));
#12572=DIRECTION('ref_axis',(0.,1.,1.15648231731787E-16));
#12573=DIRECTION('',(0.,0.,-1.));
#12574=DIRECTION('center_axis',(0.,0.,1.));
#12575=DIRECTION('ref_axis',(1.,0.,0.));
#12576=DIRECTION('center_axis',(0.,0.,-1.));
#12577=DIRECTION('ref_axis',(1.,0.,0.));
#12578=DIRECTION('center_axis',(0.,0.,1.));
#12579=DIRECTION('ref_axis',(1.,0.,0.));
#12580=DIRECTION('',(0.,0.,-1.));
#12581=DIRECTION('center_axis',(0.,0.,1.));
#12582=DIRECTION('ref_axis',(1.,0.,0.));
#12583=DIRECTION('center_axis',(0.,0.,-1.));
#12584=DIRECTION('ref_axis',(1.,0.,0.));
#12585=DIRECTION('center_axis',(0.,1.15648231731787E-16,-1.));
#12586=DIRECTION('ref_axis',(0.,1.,1.15648231731787E-16));
#12587=DIRECTION('',(0.,0.,-1.));
#12588=DIRECTION('center_axis',(0.,0.,1.));
#12589=DIRECTION('ref_axis',(1.,0.,0.));
#12590=DIRECTION('center_axis',(0.,0.,1.));
#12591=DIRECTION('ref_axis',(-1.,0.,0.));
#12592=DIRECTION('center_axis',(0.,0.,-1.));
#12593=DIRECTION('ref_axis',(-1.,0.,0.));
#12594=DIRECTION('',(0.,0.,1.));
#12595=DIRECTION('center_axis',(0.,0.,-1.));
#12596=DIRECTION('ref_axis',(-1.,0.,0.));
#12597=DIRECTION('center_axis',(0.,0.,1.));
#12598=DIRECTION('ref_axis',(-1.,0.,0.));
#12599=DIRECTION('center_axis',(0.,0.,-1.));
#12600=DIRECTION('ref_axis',(-1.,0.,0.));
#12601=DIRECTION('',(0.,0.,1.));
#12602=DIRECTION('center_axis',(0.,0.,-1.));
#12603=DIRECTION('ref_axis',(-1.,0.,0.));
#12604=DIRECTION('center_axis',(0.,0.,1.));
#12605=DIRECTION('ref_axis',(-1.,0.,0.));
#12606=DIRECTION('center_axis',(0.,0.,-1.));
#12607=DIRECTION('ref_axis',(-1.,0.,0.));
#12608=DIRECTION('',(0.,0.,1.));
#12609=DIRECTION('center_axis',(0.,0.,-1.));
#12610=DIRECTION('ref_axis',(-1.,0.,0.));
#12611=DIRECTION('center_axis',(1.,0.,0.));
#12612=DIRECTION('ref_axis',(0.,0.,1.));
#12613=DIRECTION('',(0.,1.15648231731787E-16,-1.));
#12614=DIRECTION('',(0.,1.,1.15648231731787E-16));
#12615=DIRECTION('',(0.,0.,-1.));
#12616=DIRECTION('',(0.,1.,0.));
#12617=DIRECTION('',(0.,0.,-1.));
#12618=DIRECTION('',(0.,1.,0.));
#12619=DIRECTION('',(0.,0.,1.));
#12620=DIRECTION('',(0.,1.,1.15648231731787E-16));
#12621=DIRECTION('',(0.,1.15648231731787E-16,-1.));
#12622=DIRECTION('',(0.,-1.,-1.09792625061823E-16));
#12623=DIRECTION('center_axis',(0.,1.15648231731787E-16,-1.));
#12624=DIRECTION('ref_axis',(0.,-1.,-1.15648231731787E-16));
#12625=DIRECTION('',(-1.,0.,0.));
#12626=DIRECTION('',(0.,1.,1.15648231731787E-16));
#12627=DIRECTION('center_axis',(0.,1.15648231731787E-16,-1.));
#12628=DIRECTION('ref_axis',(0.,-1.,-1.15648231731787E-16));
#12629=DIRECTION('',(-1.,0.,0.));
#12630=DIRECTION('center_axis',(0.,1.15648231731787E-16,-1.));
#12631=DIRECTION('ref_axis',(0.,-1.,-1.15648231731787E-16));
#12632=DIRECTION('',(1.,0.,0.));
#12633=DIRECTION('',(-1.,0.,0.));
#12634=DIRECTION('center_axis',(0.,1.15648231731787E-16,-1.));
#12635=DIRECTION('ref_axis',(0.,-1.,-1.15648231731787E-16));
#12636=DIRECTION('',(0.,1.,1.15648231731787E-16));
#12637=DIRECTION('center_axis',(0.,0.,-1.));
#12638=DIRECTION('ref_axis',(1.,0.,0.));
#12639=DIRECTION('',(1.,0.,0.));
#12640=DIRECTION('',(0.,-1.,0.));
#12641=DIRECTION('',(-0.977786581118157,-0.209602962253078,0.));
#12642=DIRECTION('',(-0.977786581118157,-0.209602962253079,0.));
#12643=DIRECTION('center_axis',(0.,0.,1.));
#12644=DIRECTION('ref_axis',(1.,0.,0.));
#12645=DIRECTION('',(1.,0.,0.));
#12646=DIRECTION('',(0.,1.,0.));
#12647=DIRECTION('',(0.86602540378444,0.499999999999998,0.));
#12648=DIRECTION('',(0.,-1.,0.));
#12649=DIRECTION('',(-0.866025403784439,-0.499999999999999,0.));
#12650=DIRECTION('',(-0.866025403784438,0.500000000000001,0.));
#12651=DIRECTION('',(0.,1.,0.));
#12652=DIRECTION('',(0.866025403784438,0.500000000000001,0.));
#12653=DIRECTION('',(0.866025403784439,-0.499999999999999,0.));
#12654=DIRECTION('',(0.,1.,0.));
#12655=DIRECTION('',(0.866025403784438,0.500000000000001,0.));
#12656=DIRECTION('',(0.866025403784439,-0.499999999999999,0.));
#12657=DIRECTION('',(0.,-1.,0.));
#12658=DIRECTION('',(-0.866025403784439,-0.499999999999999,0.));
#12659=DIRECTION('',(-0.866025403784438,0.500000000000001,0.));
#12660=DIRECTION('center_axis',(0.209602962253079,-0.977786581118157,0.));
#12661=DIRECTION('ref_axis',(0.977786581118157,0.209602962253079,0.));
#12662=DIRECTION('',(0.,0.,1.));
#12663=DIRECTION('',(-0.977786581118157,-0.209602962253079,0.));
#12664=DIRECTION('',(0.,0.,1.));
#12665=DIRECTION('center_axis',(0.,0.,1.));
#12666=DIRECTION('ref_axis',(0.99443113917409,0.105388374315774,0.));
#12667=DIRECTION('center_axis',(0.,0.,1.));
#12668=DIRECTION('ref_axis',(1.,0.,0.));
#12669=DIRECTION('',(0.,0.,1.));
#12670=DIRECTION('center_axis',(0.,1.,0.));
#12671=DIRECTION('ref_axis',(0.,0.,-1.));
#12672=DIRECTION('',(-1.,0.,0.));
#12673=DIRECTION('',(0.,0.,1.));
#12674=DIRECTION('',(1.,0.,0.));
#12675=DIRECTION('',(0.,0.,-1.));
#12676=DIRECTION('center_axis',(1.,0.,0.));
#12677=DIRECTION('ref_axis',(0.,0.,1.));
#12678=DIRECTION('',(0.,0.,1.));
#12679=DIRECTION('',(0.,-1.,0.));
#12680=DIRECTION('',(0.,0.,-1.));
#12681=DIRECTION('',(0.,1.15648231731787E-16,-1.));
#12682=DIRECTION('',(0.,1.,1.09792625061823E-16));
#12683=DIRECTION('',(0.,1.15648231731787E-16,-1.));
#12684=DIRECTION('center_axis',(-9.91270557701033E-17,1.,0.));
#12685=DIRECTION('ref_axis',(-1.,-9.91270557701033E-17,0.));
#12686=DIRECTION('',(0.,0.,1.));
#12687=DIRECTION('',(1.,9.91270557701033E-17,0.));
#12688=DIRECTION('center_axis',(0.,0.,-1.));
#12689=DIRECTION('ref_axis',(1.,0.,0.));
#12690=DIRECTION('center_axis',(0.,0.,1.));
#12691=DIRECTION('ref_axis',(1.,0.,0.));
#12692=DIRECTION('center_axis',(0.,0.,1.));
#12693=DIRECTION('ref_axis',(1.,0.,0.));
#12694=DIRECTION('center_axis',(0.,0.,1.));
#12695=DIRECTION('ref_axis',(-1.,0.,0.));
#12696=DIRECTION('center_axis',(0.,0.,1.));
#12697=DIRECTION('ref_axis',(-1.,0.,0.));
#12698=DIRECTION('center_axis',(-0.209602962253078,0.977786581118157,0.));
#12699=DIRECTION('ref_axis',(-0.977786581118157,-0.209602962253078,0.));
#12700=DIRECTION('',(0.,0.,-1.));
#12701=DIRECTION('',(-0.977786581118157,-0.209602962253078,0.));
#12702=DIRECTION('center_axis',(-1.,0.,0.));
#12703=DIRECTION('ref_axis',(0.,0.,-1.));
#12704=DIRECTION('',(0.,-1.,0.));
#12705=DIRECTION('',(0.,0.,-1.));
#12706=DIRECTION('center_axis',(0.,0.,1.));
#12707=DIRECTION('ref_axis',(-1.,0.,0.));
#12708=DIRECTION('',(0.,1.,0.));
#12709=DIRECTION('',(-1.,0.,0.));
#12710=DIRECTION('',(-0.86602540378444,-0.499999999999998,0.));
#12711=DIRECTION('center_axis',(0.,0.,1.));
#12712=DIRECTION('ref_axis',(-1.,0.,0.));
#12713=DIRECTION('center_axis',(0.,0.,-1.));
#12714=DIRECTION('ref_axis',(1.,0.,0.));
#12715=DIRECTION('center_axis',(0.,0.,1.));
#12716=DIRECTION('ref_axis',(-1.,0.,0.));
#12717=DIRECTION('center_axis',(0.,0.,1.));
#12718=DIRECTION('ref_axis',(-1.,0.,0.));
#12719=DIRECTION('center_axis',(-0.500000000000001,-0.866025403784438,0.));
#12720=DIRECTION('ref_axis',(0.866025403784438,-0.500000000000001,0.));
#12721=DIRECTION('',(0.,0.,1.));
#12722=DIRECTION('',(-0.866025403784438,0.500000000000001,0.));
#12723=DIRECTION('',(0.,0.,1.));
#12724=DIRECTION('center_axis',(0.499999999999999,-0.866025403784439,0.));
#12725=DIRECTION('ref_axis',(0.866025403784439,0.499999999999999,0.));
#12726=DIRECTION('',(0.,0.,1.));
#12727=DIRECTION('',(-0.866025403784439,-0.499999999999999,0.));
#12728=DIRECTION('center_axis',(1.,0.,0.));
#12729=DIRECTION('ref_axis',(0.,0.,1.));
#12730=DIRECTION('',(0.,0.,1.));
#12731=DIRECTION('',(0.,-1.,0.));
#12732=DIRECTION('center_axis',(0.499999999999999,0.866025403784439,0.));
#12733=DIRECTION('ref_axis',(-0.866025403784439,0.499999999999999,0.));
#12734=DIRECTION('',(0.,0.,1.));
#12735=DIRECTION('',(0.866025403784439,-0.499999999999999,0.));
#12736=DIRECTION('center_axis',(-0.500000000000001,0.866025403784438,0.));
#12737=DIRECTION('ref_axis',(-0.866025403784438,-0.500000000000001,0.));
#12738=DIRECTION('',(0.,0.,1.));
#12739=DIRECTION('',(0.866025403784438,0.500000000000001,0.));
#12740=DIRECTION('center_axis',(-1.,0.,0.));
#12741=DIRECTION('ref_axis',(0.,0.,-1.));
#12742=DIRECTION('',(0.,1.,0.));
#12743=DIRECTION('center_axis',(0.,0.,-1.));
#12744=DIRECTION('ref_axis',(1.,0.,0.));
#12745=DIRECTION('center_axis',(0.499999999999999,0.866025403784439,0.));
#12746=DIRECTION('ref_axis',(-0.866025403784439,0.499999999999999,0.));
#12747=DIRECTION('',(0.,0.,1.));
#12748=DIRECTION('',(0.866025403784439,-0.499999999999999,0.));
#12749=DIRECTION('',(0.,0.,1.));
#12750=DIRECTION('center_axis',(-0.500000000000001,0.866025403784438,0.));
#12751=DIRECTION('ref_axis',(-0.866025403784438,-0.500000000000001,0.));
#12752=DIRECTION('',(0.,0.,1.));
#12753=DIRECTION('',(0.866025403784438,0.500000000000001,0.));
#12754=DIRECTION('center_axis',(-1.,0.,0.));
#12755=DIRECTION('ref_axis',(0.,0.,-1.));
#12756=DIRECTION('',(0.,0.,1.));
#12757=DIRECTION('',(0.,1.,0.));
#12758=DIRECTION('center_axis',(-0.500000000000001,-0.866025403784438,0.));
#12759=DIRECTION('ref_axis',(0.866025403784438,-0.500000000000001,0.));
#12760=DIRECTION('',(0.,0.,1.));
#12761=DIRECTION('',(-0.866025403784438,0.500000000000001,0.));
#12762=DIRECTION('center_axis',(0.499999999999999,-0.866025403784439,0.));
#12763=DIRECTION('ref_axis',(0.866025403784439,0.499999999999999,0.));
#12764=DIRECTION('',(0.,0.,1.));
#12765=DIRECTION('',(-0.866025403784439,-0.499999999999999,0.));
#12766=DIRECTION('center_axis',(1.,0.,0.));
#12767=DIRECTION('ref_axis',(0.,0.,1.));
#12768=DIRECTION('',(0.,-1.,0.));
#12769=DIRECTION('center_axis',(0.,0.,1.));
#12770=DIRECTION('ref_axis',(-1.,0.,0.));
#12771=DIRECTION('center_axis',(0.,-1.,0.));
#12772=DIRECTION('ref_axis',(0.,0.,1.));
#12773=DIRECTION('',(0.,0.,-1.));
#12774=DIRECTION('center_axis',(1.,0.,0.));
#12775=DIRECTION('ref_axis',(0.,0.,1.));
#12776=DIRECTION('',(0.,0.,1.));
#12777=DIRECTION('center_axis',(-0.499999999999998,0.86602540378444,0.));
#12778=DIRECTION('ref_axis',(0.,0.,1.));
#12779=DIRECTION('center_axis',(0.,-1.09792625061823E-16,1.));
#12780=DIRECTION('ref_axis',(0.,1.,1.09792625061823E-16));
#12781=DIRECTION('',(1.,0.,0.));
#12782=DIRECTION('',(-1.,0.,0.));
#12783=DIRECTION('center_axis',(0.,1.,1.15648231731787E-16));
#12784=DIRECTION('ref_axis',(0.,1.15648231731787E-16,-1.));
#12785=DIRECTION('center_axis',(0.,-1.,-1.15648231731787E-16));
#12786=DIRECTION('ref_axis',(0.,-1.15648231731787E-16,1.));
#15853=CARTESIAN_POINT('',(0.,0.,0.));
#15854=CARTESIAN_POINT('Origin',(198.2,9.50000000000001,-9.));
#15855=CARTESIAN_POINT('',(200.2,9.50000000000001,-9.));
#15856=CARTESIAN_POINT('Origin',(198.2,9.50000000000001,-9.));
#15857=CARTESIAN_POINT('',(200.2,9.50000000000001,-3.));
#15858=CARTESIAN_POINT('',(200.2,9.50000000000001,-9.));
#15859=CARTESIAN_POINT('Origin',(198.2,9.50000000000001,-3.));
#15860=CARTESIAN_POINT('Origin',(198.2,-4.49999999999994,-9.));
#15861=CARTESIAN_POINT('',(200.2,-4.49999999999994,-9.));
#15862=CARTESIAN_POINT('Origin',(198.2,-4.49999999999994,-9.));
#15863=CARTESIAN_POINT('',(200.2,-4.49999999999994,-3.));
#15864=CARTESIAN_POINT('',(200.2,-4.49999999999994,-9.));
#15865=CARTESIAN_POINT('Origin',(198.2,-4.49999999999994,-3.));
#15866=CARTESIAN_POINT('Origin',(162.5,0.,-9.));
#15867=CARTESIAN_POINT('',(158.5,4.89858719658942E-16,-4.6));
#15868=CARTESIAN_POINT('Origin',(162.5,0.,-4.6));
#15869=CARTESIAN_POINT('',(158.5,4.89858719658942E-16,-9.));
#15870=CARTESIAN_POINT('',(158.5,4.89858719658942E-16,-9.));
#15871=CARTESIAN_POINT('Origin',(162.5,0.,-9.));
#15872=CARTESIAN_POINT('Origin',(162.5,0.,-9.));
#15873=CARTESIAN_POINT('',(160.25,2.75545529808155E-16,-1.));
#15874=CARTESIAN_POINT('Origin',(162.5,-2.31296463463574E-16,-1.));
#15875=CARTESIAN_POINT('',(160.25,2.75545529808155E-16,-4.6));
#15876=CARTESIAN_POINT('',(160.25,2.75545529808155E-16,-9.));
#15877=CARTESIAN_POINT('Origin',(162.5,0.,-4.6));
#15878=CARTESIAN_POINT('Origin',(182.5,0.,-9.));
#15879=CARTESIAN_POINT('',(178.5,4.89858719658942E-16,-4.6));
#15880=CARTESIAN_POINT('Origin',(182.5,0.,-4.6));
#15881=CARTESIAN_POINT('',(178.5,4.89858719658942E-16,-9.));
#15882=CARTESIAN_POINT('',(178.5,4.89858719658942E-16,-9.));
#15883=CARTESIAN_POINT('Origin',(182.5,0.,-9.));
#15884=CARTESIAN_POINT('Origin',(182.5,0.,-9.));
#15885=CARTESIAN_POINT('',(180.25,2.75545529808155E-16,-1.));
#15886=CARTESIAN_POINT('Origin',(182.5,-2.31296463463574E-16,-1.));
#15887=CARTESIAN_POINT('',(180.25,2.75545529808155E-16,-4.6));
#15888=CARTESIAN_POINT('',(180.25,2.75545529808155E-16,-9.));
#15889=CARTESIAN_POINT('Origin',(182.5,0.,-4.6));
#15890=CARTESIAN_POINT('Origin',(212.,2.50000000000003,-9.));
#15891=CARTESIAN_POINT('',(219.,2.50000000000003,-9.));
#15892=CARTESIAN_POINT('Origin',(212.,2.50000000000003,-9.));
#15893=CARTESIAN_POINT('',(219.,2.50000000000003,-8.));
#15894=CARTESIAN_POINT('',(219.,2.50000000000003,-9.));
#15895=CARTESIAN_POINT('Origin',(212.,2.50000000000003,-8.));
#15896=CARTESIAN_POINT('Origin',(212.,2.50000000000003,-8.));
#15897=CARTESIAN_POINT('',(222.,2.50000000000003,-8.));
#15898=CARTESIAN_POINT('Origin',(212.,2.50000000000003,-8.));
#15899=CARTESIAN_POINT('',(222.,2.50000000000003,-7.));
#15900=CARTESIAN_POINT('',(222.,2.50000000000003,-8.));
#15901=CARTESIAN_POINT('Origin',(212.,2.50000000000003,-7.));
#15902=CARTESIAN_POINT('Origin',(212.,2.50000000000003,-7.));
#15903=CARTESIAN_POINT('',(223.1,2.50000000000003,-7.));
#15904=CARTESIAN_POINT('Origin',(212.,2.50000000000003,-7.));
#15905=CARTESIAN_POINT('',(223.1,2.50000000000003,0.));
#15906=CARTESIAN_POINT('',(223.1,2.50000000000003,-7.));
#15907=CARTESIAN_POINT('Origin',(212.,2.50000000000003,0.));
#15908=CARTESIAN_POINT('Origin',(190.,0.,10.));
#15909=CARTESIAN_POINT('',(190.,-3.95,-1.));
#15910=CARTESIAN_POINT('',(190.,-3.95,-3.));
#15911=CARTESIAN_POINT('',(190.,-3.95,-1.));
#15912=CARTESIAN_POINT('',(190.,-15.,-3.));
#15913=CARTESIAN_POINT('',(190.,15.,-3.));
#15914=CARTESIAN_POINT('',(190.,-15.,0.));
#15915=CARTESIAN_POINT('',(190.,-15.,-3.));
#15916=CARTESIAN_POINT('',(190.,-13.9772819352292,0.));
#15917=CARTESIAN_POINT('',(190.,0.,0.));
#15918=CARTESIAN_POINT('',(190.,-13.9772819352292,10.));
#15919=CARTESIAN_POINT('',(190.,-13.9772819352292,10.));
#15920=CARTESIAN_POINT('',(190.,15.,10.));
#15921=CARTESIAN_POINT('',(190.,0.,10.));
#15922=CARTESIAN_POINT('',(190.,15.,-3.));
#15923=CARTESIAN_POINT('',(190.,15.,-3.));
#15924=CARTESIAN_POINT('',(190.,3.95,-3.));
#15925=CARTESIAN_POINT('',(190.,15.,-3.));
#15926=CARTESIAN_POINT('',(190.,3.95,-1.));
#15927=CARTESIAN_POINT('',(190.,3.95,-1.));
#15928=CARTESIAN_POINT('',(190.,-3.95,-1.));
#15929=CARTESIAN_POINT('Origin',(190.,15.,-3.));
#15930=CARTESIAN_POINT('',(155.,-3.94999999999999,-3.));
#15931=CARTESIAN_POINT('',(155.,-3.95,-3.));
#15932=CARTESIAN_POINT('',(155.,-13.,-3.));
#15933=CARTESIAN_POINT('',(155.,15.,-3.));
#15934=CARTESIAN_POINT('',(157.,-15.,-3.));
#15935=CARTESIAN_POINT('Origin',(157.,-13.,-3.));
#15936=CARTESIAN_POINT('',(190.,-15.,-3.));
#15937=CARTESIAN_POINT('Origin',(190.,15.,-3.));
#15938=CARTESIAN_POINT('',(155.,3.95,-3.));
#15939=CARTESIAN_POINT('',(155.,3.95,-3.));
#15940=CARTESIAN_POINT('',(157.,15.,-3.));
#15941=CARTESIAN_POINT('',(190.,15.,-3.));
#15942=CARTESIAN_POINT('',(155.,13.,-3.));
#15943=CARTESIAN_POINT('Origin',(157.,13.,-3.));
#15944=CARTESIAN_POINT('',(155.,15.,-3.));
#15945=CARTESIAN_POINT('Origin',(0.,0.,0.));
#15946=CARTESIAN_POINT('',(195.,13.,0.));
#15947=CARTESIAN_POINT('',(203.5,13.,0.));
#15948=CARTESIAN_POINT('',(190.,13.,0.));
#15949=CARTESIAN_POINT('',(195.,-12.9054582556007,0.));
#15950=CARTESIAN_POINT('',(195.,0.,0.));
#15951=CARTESIAN_POINT('',(11.2119478347524,-52.3031355243012,0.));
#15952=CARTESIAN_POINT('',(214.620037028164,-9.72233226397694,0.));
#15953=CARTESIAN_POINT('',(11.4215507970056,-53.2809221054195,0.));
#15954=CARTESIAN_POINT('',(212.,15.,0.));
#15955=CARTESIAN_POINT('Origin',(212.,2.50000000000003,0.));
#15956=CARTESIAN_POINT('',(205.,15.,0.));
#15957=CARTESIAN_POINT('',(0.,15.,0.));
#15958=CARTESIAN_POINT('',(205.,13.8660254037845,0.));
#15959=CARTESIAN_POINT('',(205.,13.,0.));
#15960=CARTESIAN_POINT('',(45.2458348754007,-78.3680848350663,0.));
#15961=CARTESIAN_POINT('',(201.2,11.2320508075689,0.));
#15962=CARTESIAN_POINT('',(201.2,7.76794919243114,0.));
#15963=CARTESIAN_POINT('',(201.2,11.2320508075689,0.));
#15964=CARTESIAN_POINT('',(198.2,6.03589838486225,0.));
#15965=CARTESIAN_POINT('',(201.2,7.76794919243114,0.));
#15966=CARTESIAN_POINT('',(195.2,7.76794919243112,0.));
#15967=CARTESIAN_POINT('',(198.2,6.03589838486225,0.));
#15968=CARTESIAN_POINT('',(195.2,11.2320508075689,0.));
#15969=CARTESIAN_POINT('',(195.2,7.76794919243112,0.));
#15970=CARTESIAN_POINT('',(198.2,12.9641016151378,0.));
#15971=CARTESIAN_POINT('',(195.2,11.2320508075689,0.));
#15972=CARTESIAN_POINT('',(198.2,12.9641016151378,0.));
#15973=CARTESIAN_POINT('',(195.2,-6.23205080756882,0.));
#15974=CARTESIAN_POINT('',(195.2,-2.76794919243105,0.));
#15975=CARTESIAN_POINT('',(195.2,-2.76794919243105,0.));
#15976=CARTESIAN_POINT('',(198.2,-1.03589838486218,0.));
#15977=CARTESIAN_POINT('',(198.2,-1.03589838486218,0.));
#15978=CARTESIAN_POINT('',(201.2,-2.76794919243107,0.));
#15979=CARTESIAN_POINT('',(201.2,-2.76794919243107,0.));
#15980=CARTESIAN_POINT('',(201.2,-6.23205080756883,0.));
#15981=CARTESIAN_POINT('',(201.2,-6.23205080756883,0.));
#15982=CARTESIAN_POINT('',(198.2,-7.9641016151377,0.));
#15983=CARTESIAN_POINT('',(198.2,-7.9641016151377,0.));
#15984=CARTESIAN_POINT('',(195.2,-6.23205080756882,0.));
#15985=CARTESIAN_POINT('Origin',(11.4215507970056,-53.2809221054195,-9.));
#15986=CARTESIAN_POINT('',(190.,-15.,-9.));
#15987=CARTESIAN_POINT('',(190.,-15.,-9.));
#15988=CARTESIAN_POINT('',(214.620037028164,-9.72233226397694,-9.));
#15989=CARTESIAN_POINT('',(11.4215507970056,-53.2809221054195,-9.));
#15990=CARTESIAN_POINT('',(214.620037028164,-9.72233226397694,-9.));
#15991=CARTESIAN_POINT('Origin',(212.,2.50000000000003,-9.));
#15992=CARTESIAN_POINT('',(212.,15.,-9.));
#15993=CARTESIAN_POINT('Origin',(212.,2.50000000000003,-9.));
#15994=CARTESIAN_POINT('',(212.,15.,-9.));
#15995=CARTESIAN_POINT('Origin',(0.,15.,-9.));
#15996=CARTESIAN_POINT('',(205.,15.,10.));
#15997=CARTESIAN_POINT('',(190.,15.,10.));
#15998=CARTESIAN_POINT('',(205.,15.,0.));
#15999=CARTESIAN_POINT('',(157.,15.,-9.));
#16000=CARTESIAN_POINT('',(0.,15.,-9.));
#16001=CARTESIAN_POINT('',(157.,15.,-9.));
#16002=CARTESIAN_POINT('Origin',(155.,0.,-9.));
#16003=CARTESIAN_POINT('',(155.,13.,-9.));
#16004=CARTESIAN_POINT('',(155.,13.,0.));
#16005=CARTESIAN_POINT('',(155.,-13.,-9.));
#16006=CARTESIAN_POINT('',(155.,0.,-9.));
#16007=CARTESIAN_POINT('',(155.,-13.,-9.));
#16008=CARTESIAN_POINT('',(155.,-3.95,-1.));
#16009=CARTESIAN_POINT('',(155.,-3.95,-1.));
#16010=CARTESIAN_POINT('',(155.,3.95,-1.));
#16011=CARTESIAN_POINT('',(155.,-3.95,-1.));
#16012=CARTESIAN_POINT('',(155.,3.95,-1.));
#16013=CARTESIAN_POINT('Origin',(1.48690583655155E-15,-15.,-9.));
#16014=CARTESIAN_POINT('',(157.,-15.,-9.));
#16015=CARTESIAN_POINT('',(157.,-15.,-9.));
#16016=CARTESIAN_POINT('',(1.48690583655155E-15,-15.,-9.));
#16017=CARTESIAN_POINT('Origin',(0.,0.,-9.));
#16018=CARTESIAN_POINT('Origin',(157.,13.,-9.));
#16019=CARTESIAN_POINT('Origin',(157.,-13.,-9.));
#16020=CARTESIAN_POINT('Origin',(212.,2.50000000000003,-7.));
#16021=CARTESIAN_POINT('Origin',(212.,2.50000000000003,-8.));
#16022=CARTESIAN_POINT('Origin',(11.2119478347524,-52.3031355243012,10.));
#16023=CARTESIAN_POINT('',(195.,-12.9054582556007,10.));
#16024=CARTESIAN_POINT('',(195.,-12.9054582556007,10.));
#16025=CARTESIAN_POINT('',(11.2119478347524,-52.3031355243012,10.));
#16026=CARTESIAN_POINT('Origin',(195.,0.,10.));
#16027=CARTESIAN_POINT('',(195.,13.,10.));
#16028=CARTESIAN_POINT('',(195.,0.,10.));
#16029=CARTESIAN_POINT('',(195.,13.,10.));
#16030=CARTESIAN_POINT('Origin',(0.,0.,10.));
#16031=CARTESIAN_POINT('',(205.,13.8660254037845,10.));
#16032=CARTESIAN_POINT('',(205.,13.,10.));
#16033=CARTESIAN_POINT('',(203.5,13.,10.));
#16034=CARTESIAN_POINT('',(190.,13.,10.));
#16035=CARTESIAN_POINT('',(45.2458348754007,-78.3680848350663,10.));
#16036=CARTESIAN_POINT('Origin',(157.,-13.,-9.));
#16037=CARTESIAN_POINT('Origin',(157.,13.,-9.));
#16038=CARTESIAN_POINT('Origin',(184.75,0.,-4.6));
#16039=CARTESIAN_POINT('Origin',(164.75,0.,-4.6));
#16040=CARTESIAN_POINT('Origin',(195.2,-6.23205080756882,-3.));
#16041=CARTESIAN_POINT('',(198.2,-7.9641016151377,-3.));
#16042=CARTESIAN_POINT('',(198.2,-7.9641016151377,-3.));
#16043=CARTESIAN_POINT('',(195.2,-6.23205080756882,-3.));
#16044=CARTESIAN_POINT('',(195.2,-6.23205080756882,-3.));
#16045=CARTESIAN_POINT('',(195.2,-6.23205080756882,-3.));
#16046=CARTESIAN_POINT('Origin',(198.2,-7.9641016151377,-3.));
#16047=CARTESIAN_POINT('',(201.2,-6.23205080756883,-3.));
#16048=CARTESIAN_POINT('',(201.2,-6.23205080756883,-3.));
#16049=CARTESIAN_POINT('',(198.2,-7.9641016151377,-3.));
#16050=CARTESIAN_POINT('Origin',(201.2,-6.23205080756883,-3.));
#16051=CARTESIAN_POINT('',(201.2,-2.76794919243107,-3.));
#16052=CARTESIAN_POINT('',(201.2,-2.76794919243107,-3.));
#16053=CARTESIAN_POINT('',(201.2,-6.23205080756883,-3.));
#16054=CARTESIAN_POINT('Origin',(201.2,-2.76794919243107,-3.));
#16055=CARTESIAN_POINT('',(198.2,-1.03589838486218,-3.));
#16056=CARTESIAN_POINT('',(198.2,-1.03589838486218,-3.));
#16057=CARTESIAN_POINT('',(201.2,-2.76794919243107,-3.));
#16058=CARTESIAN_POINT('Origin',(198.2,-1.03589838486218,-3.));
#16059=CARTESIAN_POINT('',(195.2,-2.76794919243105,-3.));
#16060=CARTESIAN_POINT('',(195.2,-2.76794919243105,-3.));
#16061=CARTESIAN_POINT('',(198.2,-1.03589838486218,-3.));
#16062=CARTESIAN_POINT('Origin',(195.2,-2.76794919243105,-3.));
#16063=CARTESIAN_POINT('',(195.2,-2.76794919243105,-3.));
#16064=CARTESIAN_POINT('Origin',(0.,0.,-3.));
#16065=CARTESIAN_POINT('Origin',(198.2,12.9641016151378,-3.));
#16066=CARTESIAN_POINT('',(198.2,12.9641016151378,-3.));
#16067=CARTESIAN_POINT('',(198.2,12.9641016151378,-3.));
#16068=CARTESIAN_POINT('',(201.2,11.2320508075689,-3.));
#16069=CARTESIAN_POINT('',(198.2,12.9641016151378,-3.));
#16070=CARTESIAN_POINT('',(201.2,11.2320508075689,-3.));
#16071=CARTESIAN_POINT('Origin',(195.2,11.2320508075689,-3.));
#16072=CARTESIAN_POINT('',(195.2,11.2320508075689,-3.));
#16073=CARTESIAN_POINT('',(195.2,11.2320508075689,-3.));
#16074=CARTESIAN_POINT('',(195.2,11.2320508075689,-3.));
#16075=CARTESIAN_POINT('Origin',(195.2,7.76794919243112,-3.));
#16076=CARTESIAN_POINT('',(195.2,7.76794919243112,-3.));
#16077=CARTESIAN_POINT('',(195.2,7.76794919243112,-3.));
#16078=CARTESIAN_POINT('',(195.2,7.76794919243112,-3.));
#16079=CARTESIAN_POINT('Origin',(198.2,6.03589838486225,-3.));
#16080=CARTESIAN_POINT('',(198.2,6.03589838486225,-3.));
#16081=CARTESIAN_POINT('',(198.2,6.03589838486225,-3.));
#16082=CARTESIAN_POINT('',(198.2,6.03589838486225,-3.));
#16083=CARTESIAN_POINT('Origin',(201.2,7.76794919243114,-3.));
#16084=CARTESIAN_POINT('',(201.2,7.76794919243114,-3.));
#16085=CARTESIAN_POINT('',(201.2,7.76794919243114,-3.));
#16086=CARTESIAN_POINT('',(201.2,7.76794919243114,-3.));
#16087=CARTESIAN_POINT('Origin',(201.2,11.2320508075689,-3.));
#16088=CARTESIAN_POINT('',(201.2,11.2320508075689,-3.));
#16089=CARTESIAN_POINT('Origin',(0.,0.,-3.));
#16090=CARTESIAN_POINT('Origin',(0.,13.,0.));
#16091=CARTESIAN_POINT('',(203.5,13.,0.));
#16092=CARTESIAN_POINT('Origin',(205.,13.,0.));
#16093=CARTESIAN_POINT('',(205.,13.8660254037845,0.));
#16094=CARTESIAN_POINT('Origin',(205.,13.8660254037845,0.));
#16095=CARTESIAN_POINT('Origin',(0.,9.80814117218957E-17,-1.));
#16096=CARTESIAN_POINT('',(155.,3.95,-1.));
#16097=CARTESIAN_POINT('',(155.,-3.95,-1.));
#16098=CARTESIAN_POINT('Origin',(155.,-3.95,-1.));
#16099=CARTESIAN_POINT('Origin',(155.,3.95,-1.));
#18834=UNCERTAINTY_MEASURE_WITH_UNIT(LENGTH_MEASURE(0.01),#18868,
'DISTANCE_ACCURACY_VALUE',
'Maximum model space distance between geometric entities at asserted c
onnectivities');
#18849=UNCERTAINTY_MEASURE_WITH_UNIT(LENGTH_MEASURE(0.01),#18868,
'DISTANCE_ACCURACY_VALUE',
'Maximum model space distance between geometric entities at asserted c
onnectivities');
#18852=(
GEOMETRIC_REPRESENTATION_CONTEXT(3)
GLOBAL_UNCERTAINTY_ASSIGNED_CONTEXT((#18834))
GLOBAL_UNIT_ASSIGNED_CONTEXT((#18868,#18870,#18871))
REPRESENTATION_CONTEXT('','3D')
);
#18867=(
GEOMETRIC_REPRESENTATION_CONTEXT(3)
GLOBAL_UNCERTAINTY_ASSIGNED_CONTEXT((#18849))
GLOBAL_UNIT_ASSIGNED_CONTEXT((#18868,#18870,#18871))
REPRESENTATION_CONTEXT('','3D')
);
#18868=(
LENGTH_UNIT()
NAMED_UNIT(*)
SI_UNIT(.MILLI.,.METRE.)
);
#18870=(
NAMED_UNIT(*)
PLANE_ANGLE_UNIT()
SI_UNIT($,.RADIAN.)
);
#18871=(
NAMED_UNIT(*)
SI_UNIT($,.STERADIAN.)
SOLID_ANGLE_UNIT()
);
#18874=SHAPE_DEFINITION_REPRESENTATION(#18891,#18936);
#18891=PRODUCT_DEFINITION_SHAPE('',$,#18954);
#18936=SHAPE_REPRESENTATION('',(#11233),#18852);
#18951=PRODUCT_DEFINITION_CONTEXT('part definition',#19004,'design');
#18954=PRODUCT_DEFINITION('Drive End Bracket 2','Drive End Bracket 2',#18971,
#18951);
#18971=PRODUCT_DEFINITION_FORMATION('',$,#19008);
#19004=APPLICATION_CONTEXT(
'Core Data for Automotive Mechanical Design Process');
#19005=PRODUCT_CONTEXT('part definition',#19004,'mechanical');
#19008=PRODUCT('Drive End Bracket 2','Drive End Bracket 2',$,(#19005));
#19024=PRESENTATION_STYLE_ASSIGNMENT((#19030));
#19030=SURFACE_STYLE_USAGE(.BOTH.,#19036);
#19036=SURFACE_SIDE_STYLE('',(#19042));
#19042=SURFACE_STYLE_FILL_AREA(#19048);
#19048=FILL_AREA_STYLE('Opaque(20,51,87)',(#19054));
#19054=FILL_AREA_STYLE_COLOUR('Opaque(20,51,87)',#19060);
#19060=COLOUR_RGB('Opaque(20,51,87)',0.0784313725490196,0.2,0.341176470588235);
ENDSEC;
END-ISO-10303-21;
